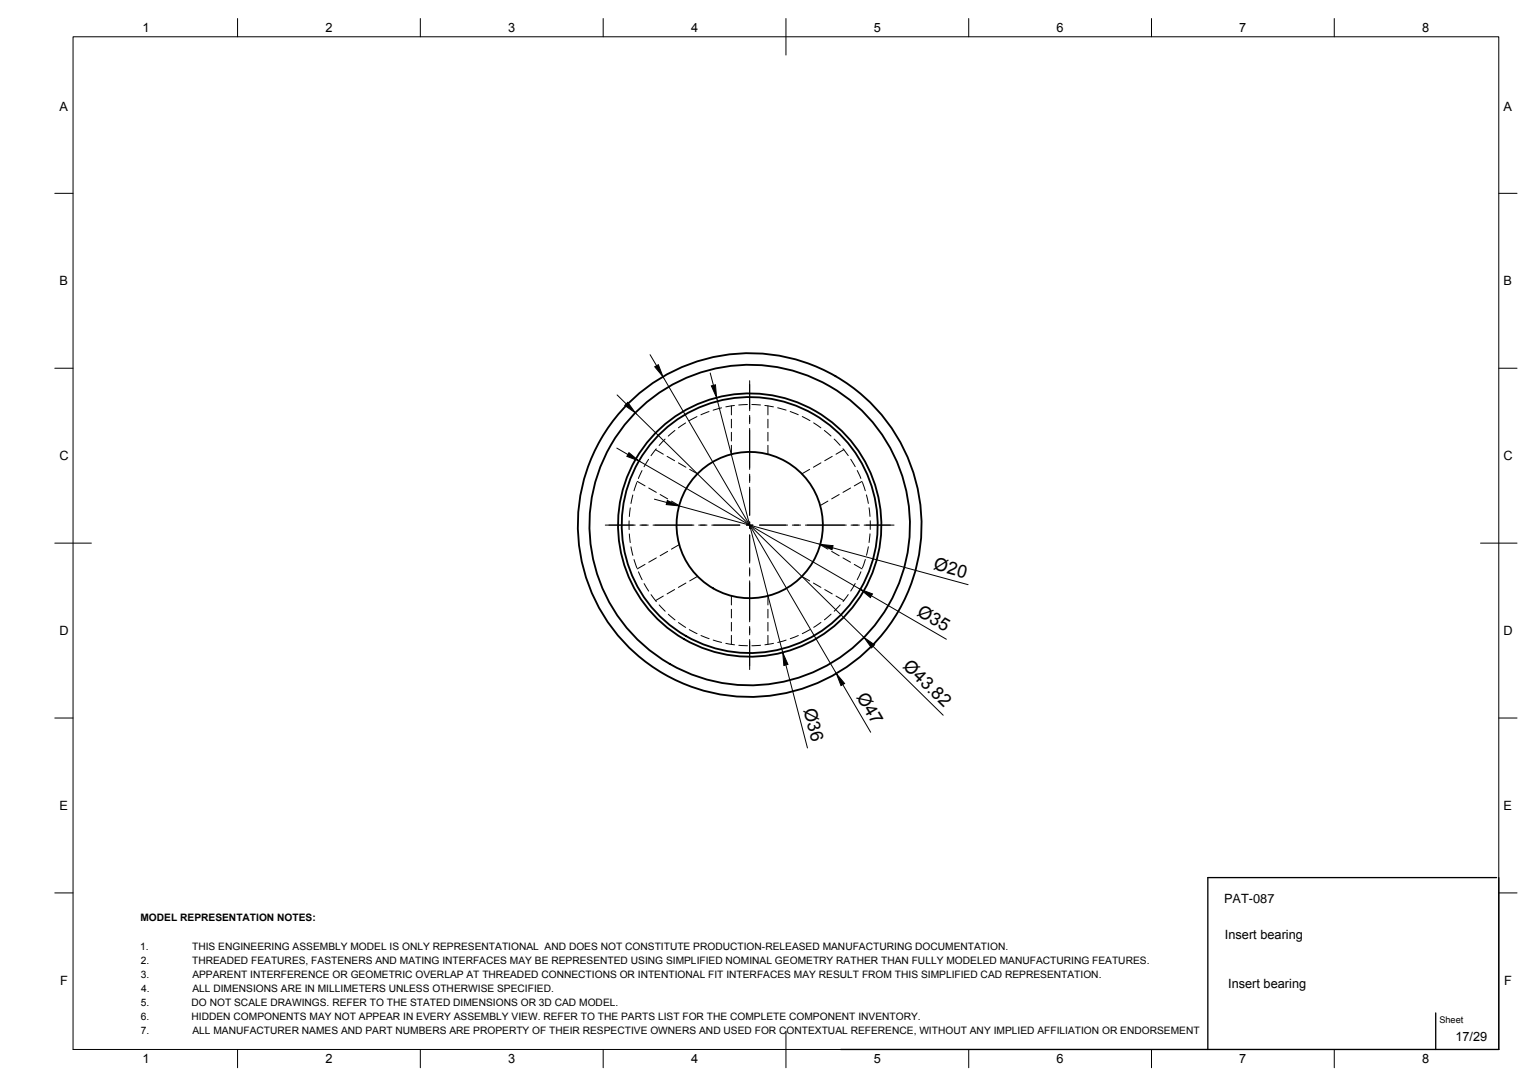
ISO-10303-21;
HEADER;
/* Generated by software containing ST-Developer
 * from STEP Tools, Inc. (www.steptools.com) 
 */

FILE_DESCRIPTION(
/* description */ ('Rigid flange shaft coupling assembly'),
/* implementation_level */ '2;1');

FILE_NAME(
/* name */ 'Insert bearing.step',
/* time_stamp */ '2026-10-27T10:47:16-07:00',
/* author */ (''),
/* organization */ (''),
/* preprocessor_version */ 'ST-DEVELOPER v20.2',
/* originating_system */ 'Autodesk Translation Framework v15.17.0.0',
/* authorisation */ '');

FILE_SCHEMA (('AUTOMOTIVE_DESIGN { 1 0 10303 214 3 1 1 }'));
ENDSEC;

DATA;
#10=MECHANICAL_DESIGN_GEOMETRIC_PRESENTATION_REPRESENTATION('',(#408,#409),#9141);
#300=B_SPLINE_CURVE_WITH_KNOTS('',3,(#7504,#7505,#7506,#7507,#7508,#7509,
#7510,#7511,#7512,#7513),.UNSPECIFIED.,.F.,.F.,(4,2,2,2,4),(1.13193471301885,
1.22626174930539,1.32058878559194,1.41491753480854,1.50924628402513),
 .UNSPECIFIED.);
#301=B_SPLINE_CURVE_WITH_KNOTS('',3,(#7515,#7516,#7517,#7518,#7519,#7520,
#7521,#7522,#7523,#7524,#7525,#7526,#7527,#7528,#7529,#7530,#7531,#7532),
 .UNSPECIFIED.,.F.,.F.,(4,2,2,2,2,2,2,2,4),(0.377311571006283,0.471638607292829,
0.565965643579376,0.66029439279597,0.754623142012565,0.84895189122916,0.943280640445754,
1.0376076767323,1.13193471301885),.UNSPECIFIED.);
#302=B_SPLINE_CURVE_WITH_KNOTS('',3,(#7533,#7534,#7535,#7536,#7537,#7538,
#7539,#7540,#7541,#7542),.UNSPECIFIED.,.F.,.F.,(4,2,2,2,4),(1.50924628402513,
1.60357503324173,1.69790378245832,1.79223081874487,1.88655785503141),
 .UNSPECIFIED.);
#303=B_SPLINE_CURVE_WITH_KNOTS('',3,(#7545,#7546,#7547,#7548,#7549,#7550,
#7551,#7552,#7553,#7554,#7555,#7556,#7557,#7558,#7559,#7560,#7561,#7562,
#7563,#7564,#7565,#7566,#7567,#7568,#7569,#7570,#7571,#7572,#7573,#7574,
#7575,#7576,#7577,#7578),.UNSPECIFIED.,.T.,.F.,(4,2,2,2,2,2,2,2,2,2,2,2,
2,2,2,2,4),(0.,0.0946120580087934,0.189224116017587,0.283822945575014,0.378421775132442,
0.47302060468987,0.567619434247297,0.662231492256091,0.756843550264884,
0.851455608273677,0.94606766628247,1.0406664958399,1.13526532539733,1.22986415495475,
1.32446298451218,1.41907504252097,1.51368710052977),.UNSPECIFIED.);
#304=B_SPLINE_CURVE_WITH_KNOTS('',3,(#7581,#7582,#7583,#7584,#7585,#7586,
#7587,#7588,#7589,#7590,#7591,#7592,#7593,#7594,#7595,#7596,#7597,#7598,
#7599,#7600,#7601,#7602,#7603,#7604,#7605,#7606,#7607,#7608,#7609,#7610,
#7611,#7612,#7613,#7614),.UNSPECIFIED.,.T.,.F.,(4,2,2,2,2,2,2,2,2,2,2,2,
2,2,2,2,4),(0.,0.0946120580087934,0.189224116017587,0.283822945575014,0.378421775132442,
0.47302060468987,0.567619434247297,0.66223149225609,0.756843550264884,0.851455608273677,
0.94606766628247,1.0406664958399,1.13526532539733,1.22986415495475,1.32446298451218,
1.41907504252097,1.51368710052977),.UNSPECIFIED.);
#305=B_SPLINE_CURVE_WITH_KNOTS('',3,(#7618,#7619,#7620,#7621,#7622,#7623,
#7624,#7625,#7626,#7627),.UNSPECIFIED.,.F.,.F.,(4,2,2,2,4),(1.13193471301885,
1.22626174930539,1.32058878559194,1.41491753480854,1.50924628402513),
 .UNSPECIFIED.);
#306=B_SPLINE_CURVE_WITH_KNOTS('',3,(#7629,#7630,#7631,#7632,#7633,#7634,
#7635,#7636,#7637,#7638,#7639,#7640,#7641,#7642,#7643,#7644,#7645,#7646),
 .UNSPECIFIED.,.F.,.F.,(4,2,2,2,2,2,2,2,4),(0.377311571006283,0.47163860729283,
0.565965643579376,0.660294392795971,0.754623142012565,0.84895189122916,
0.943280640445755,1.0376076767323,1.13193471301885),.UNSPECIFIED.);
#307=B_SPLINE_CURVE_WITH_KNOTS('',3,(#7647,#7648,#7649,#7650,#7651,#7652,
#7653,#7654,#7655,#7656),.UNSPECIFIED.,.F.,.F.,(4,2,2,2,4),(1.50924628402513,
1.60357503324173,1.69790378245832,1.79223081874487,1.88655785503141),
 .UNSPECIFIED.);
#308=B_SPLINE_CURVE_WITH_KNOTS('',3,(#7665,#7666,#7667,#7668,#7669,#7670,
#7671,#7672,#7673,#7674,#7675,#7676,#7677,#7678,#7679,#7680,#7681,#7682),
 .UNSPECIFIED.,.F.,.F.,(4,2,2,2,2,2,2,2,4),(0.377311571006282,0.471638607292829,
0.565965643579376,0.660294392795971,0.754623142012565,0.84895189122916,
0.943280640445754,1.0376076767323,1.13193471301885),.UNSPECIFIED.);
#309=B_SPLINE_CURVE_WITH_KNOTS('',3,(#7684,#7685,#7686,#7687,#7688,#7689,
#7690,#7691,#7692,#7693),.UNSPECIFIED.,.F.,.F.,(4,2,2,2,4),(1.13193471301885,
1.22626174930539,1.32058878559194,1.41491753480854,1.50924628402513),
 .UNSPECIFIED.);
#310=B_SPLINE_CURVE_WITH_KNOTS('',3,(#7694,#7695,#7696,#7697,#7698,#7699,
#7700,#7701,#7702,#7703),.UNSPECIFIED.,.F.,.F.,(4,2,2,2,4),(1.50924628402513,
1.60357503324172,1.69790378245832,1.79223081874487,1.88655785503141),
 .UNSPECIFIED.);
#311=B_SPLINE_CURVE_WITH_KNOTS('',3,(#7706,#7707,#7708,#7709,#7710,#7711,
#7712,#7713,#7714,#7715,#7716,#7717,#7718,#7719,#7720,#7721,#7722,#7723),
 .UNSPECIFIED.,.F.,.F.,(4,2,2,2,2,2,2,2,4),(0.377311571006283,0.47163860729283,
0.565965643579376,0.660294392795971,0.754623142012565,0.84895189122916,
0.943280640445754,1.0376076767323,1.13193471301885),.UNSPECIFIED.);
#312=B_SPLINE_CURVE_WITH_KNOTS('',3,(#7725,#7726,#7727,#7728,#7729,#7730,
#7731,#7732,#7733,#7734),.UNSPECIFIED.,.F.,.F.,(4,2,2,2,4),(1.13193471301885,
1.22626174930539,1.32058878559194,1.41491753480854,1.50924628402513),
 .UNSPECIFIED.);
#313=B_SPLINE_CURVE_WITH_KNOTS('',3,(#7735,#7736,#7737,#7738,#7739,#7740,
#7741,#7742,#7743,#7744),.UNSPECIFIED.,.F.,.F.,(4,2,2,2,4),(1.50924628402513,
1.60357503324173,1.69790378245832,1.79223081874487,1.88655785503141),
 .UNSPECIFIED.);
#314=B_SPLINE_CURVE_WITH_KNOTS('',3,(#7747,#7748,#7749,#7750,#7751,#7752,
#7753,#7754,#7755,#7756,#7757,#7758,#7759,#7760,#7761,#7762,#7763,#7764),
 .UNSPECIFIED.,.F.,.F.,(4,2,2,2,2,2,2,2,4),(0.377311571006282,0.471638607292829,
0.565965643579376,0.66029439279597,0.754623142012565,0.84895189122916,0.943280640445754,
1.0376076767323,1.13193471301885),.UNSPECIFIED.);
#315=B_SPLINE_CURVE_WITH_KNOTS('',3,(#7766,#7767,#7768,#7769,#7770,#7771,
#7772,#7773,#7774,#7775),.UNSPECIFIED.,.F.,.F.,(4,2,2,2,4),(1.13193471301885,
1.22626174930539,1.32058878559194,1.41491753480854,1.50924628402513),
 .UNSPECIFIED.);
#316=B_SPLINE_CURVE_WITH_KNOTS('',3,(#7776,#7777,#7778,#7779,#7780,#7781,
#7782,#7783,#7784,#7785),.UNSPECIFIED.,.F.,.F.,(4,2,2,2,4),(1.50924628402513,
1.60357503324172,1.69790378245832,1.79223081874487,1.88655785503141),
 .UNSPECIFIED.);
#317=B_SPLINE_CURVE_WITH_KNOTS('',3,(#7788,#7789,#7790,#7791,#7792,#7793,
#7794,#7795,#7796,#7797,#7798,#7799,#7800,#7801,#7802,#7803,#7804,#7805),
 .UNSPECIFIED.,.F.,.F.,(4,2,2,2,2,2,2,2,4),(0.377311571006283,0.471638607292829,
0.565965643579376,0.660294392795971,0.754623142012565,0.84895189122916,
0.943280640445755,1.0376076767323,1.13193471301885),.UNSPECIFIED.);
#318=B_SPLINE_CURVE_WITH_KNOTS('',3,(#7807,#7808,#7809,#7810,#7811,#7812,
#7813,#7814,#7815,#7816),.UNSPECIFIED.,.F.,.F.,(4,2,2,2,4),(1.13193471301885,
1.22626174930539,1.32058878559194,1.41491753480854,1.50924628402513),
 .UNSPECIFIED.);
#319=B_SPLINE_CURVE_WITH_KNOTS('',3,(#7817,#7818,#7819,#7820,#7821,#7822,
#7823,#7824,#7825,#7826),.UNSPECIFIED.,.F.,.F.,(4,2,2,2,4),(1.50924628402513,
1.60357503324172,1.69790378245832,1.79223081874487,1.88655785503141),
 .UNSPECIFIED.);
#320=B_SPLINE_CURVE_WITH_KNOTS('',3,(#7830,#7831,#7832,#7833,#7834,#7835,
#7836,#7837,#7838,#7839,#7840,#7841,#7842,#7843,#7844,#7845,#7846,#7847,
#7848,#7849,#7850,#7851,#7852,#7853,#7854,#7855,#7856,#7857,#7858,#7859,
#7860,#7861,#7862,#7863),.UNSPECIFIED.,.T.,.F.,(4,2,2,2,2,2,2,2,2,2,2,2,
2,2,2,2,4),(0.,0.0946120580087934,0.189224116017587,0.283822945575014,0.378421775132442,
0.47302060468987,0.567619434247297,0.66223149225609,0.756843550264884,0.851455608273677,
0.94606766628247,1.0406664958399,1.13526532539733,1.22986415495475,1.32446298451218,
1.41907504252097,1.51368710052977),.UNSPECIFIED.);
#321=B_SPLINE_CURVE_WITH_KNOTS('',3,(#7866,#7867,#7868,#7869,#7870,#7871,
#7872,#7873,#7874,#7875,#7876,#7877,#7878,#7879,#7880,#7881,#7882,#7883,
#7884,#7885,#7886,#7887,#7888,#7889,#7890,#7891,#7892,#7893,#7894,#7895,
#7896,#7897,#7898,#7899),.UNSPECIFIED.,.T.,.F.,(4,2,2,2,2,2,2,2,2,2,2,2,
2,2,2,2,4),(0.,0.0946120580087934,0.189224116017587,0.283822945575014,0.378421775132442,
0.47302060468987,0.567619434247297,0.66223149225609,0.756843550264884,0.851455608273677,
0.94606766628247,1.0406664958399,1.13526532539733,1.22986415495475,1.32446298451218,
1.41907504252097,1.51368710052977),.UNSPECIFIED.);
#322=B_SPLINE_CURVE_WITH_KNOTS('',3,(#7904,#7905,#7906,#7907,#7908,#7909,
#7910,#7911,#7912,#7913,#7914,#7915,#7916,#7917,#7918,#7919,#7920,#7921,
#7922,#7923,#7924,#7925,#7926,#7927,#7928,#7929,#7930,#7931,#7932,#7933,
#7934,#7935,#7936,#7937),.UNSPECIFIED.,.T.,.F.,(4,2,2,2,2,2,2,2,2,2,2,2,
2,2,2,2,4),(0.,0.0946120580087934,0.189224116017587,0.283822945575014,0.378421775132442,
0.47302060468987,0.567619434247297,0.66223149225609,0.756843550264884,0.851455608273677,
0.94606766628247,1.0406664958399,1.13526532539733,1.22986415495475,1.32446298451218,
1.41907504252097,1.51368710052977),.UNSPECIFIED.);
#323=B_SPLINE_CURVE_WITH_KNOTS('',3,(#7940,#7941,#7942,#7943,#7944,#7945,
#7946,#7947,#7948,#7949,#7950,#7951,#7952,#7953,#7954,#7955,#7956,#7957,
#7958,#7959,#7960,#7961,#7962,#7963,#7964,#7965,#7966,#7967,#7968,#7969,
#7970,#7971,#7972,#7973),.UNSPECIFIED.,.T.,.F.,(4,2,2,2,2,2,2,2,2,2,2,2,
2,2,2,2,4),(0.,0.0946120580087934,0.189224116017587,0.283822945575014,0.378421775132442,
0.47302060468987,0.567619434247297,0.66223149225609,0.756843550264884,0.851455608273677,
0.94606766628247,1.0406664958399,1.13526532539733,1.22986415495475,1.32446298451218,
1.41907504252097,1.51368710052977),.UNSPECIFIED.);
#341=SPHERICAL_SURFACE('',#5250,2.35);
#352=SHAPE_REPRESENTATION_RELATIONSHIP('SRR','None',#9287,#380);
#380=ADVANCED_BREP_SHAPE_REPRESENTATION('',(#437,#438),#9122);
#408=STYLED_ITEM('',(#9500),#437);
#409=STYLED_ITEM('',(#9500),#438);
#437=MANIFOLD_SOLID_BREP('Body1',#4762);
#438=MANIFOLD_SOLID_BREP('Body2',#4763);
#495=FACE_BOUND('',#1143,.T.);
#496=FACE_BOUND('',#1145,.T.);
#497=FACE_BOUND('',#1146,.T.);
#498=FACE_BOUND('',#1148,.T.);
#499=FACE_BOUND('',#1152,.T.);
#500=FACE_BOUND('',#1153,.T.);
#501=FACE_BOUND('',#1154,.T.);
#502=FACE_BOUND('',#1155,.T.);
#503=FACE_BOUND('',#1156,.T.);
#504=FACE_BOUND('',#1157,.T.);
#505=FACE_BOUND('',#1163,.T.);
#506=FACE_BOUND('',#1165,.T.);
#507=FACE_BOUND('',#1168,.T.);
#508=FACE_BOUND('',#1170,.T.);
#509=FACE_BOUND('',#1171,.T.);
#510=FACE_BOUND('',#1172,.T.);
#511=FACE_BOUND('',#1173,.T.);
#512=FACE_BOUND('',#1174,.T.);
#513=FACE_BOUND('',#1175,.T.);
#627=PLANE('',#5248);
#628=PLANE('',#5253);
#629=PLANE('',#5263);
#630=PLANE('',#5265);
#631=PLANE('',#5269);
#827=FACE_OUTER_BOUND('',#1141,.T.);
#828=FACE_OUTER_BOUND('',#1142,.T.);
#829=FACE_OUTER_BOUND('',#1144,.T.);
#830=FACE_OUTER_BOUND('',#1147,.T.);
#831=FACE_OUTER_BOUND('',#1149,.T.);
#832=FACE_OUTER_BOUND('',#1150,.T.);
#833=FACE_OUTER_BOUND('',#1151,.T.);
#834=FACE_OUTER_BOUND('',#1158,.T.);
#835=FACE_OUTER_BOUND('',#1159,.T.);
#836=FACE_OUTER_BOUND('',#1160,.T.);
#837=FACE_OUTER_BOUND('',#1161,.T.);
#838=FACE_OUTER_BOUND('',#1162,.T.);
#839=FACE_OUTER_BOUND('',#1164,.T.);
#840=FACE_OUTER_BOUND('',#1166,.T.);
#841=FACE_OUTER_BOUND('',#1167,.T.);
#842=FACE_OUTER_BOUND('',#1169,.T.);
#1141=EDGE_LOOP('',(#3605,#3606,#3607,#3608));
#1142=EDGE_LOOP('',(#3609));
#1143=EDGE_LOOP('',(#3610));
#1144=EDGE_LOOP('',(#3611,#3612));
#1145=EDGE_LOOP('',(#3613));
#1146=EDGE_LOOP('',(#3614));
#1147=EDGE_LOOP('',(#3615));
#1148=EDGE_LOOP('',(#3616));
#1149=EDGE_LOOP('',(#3617,#3618,#3619,#3620,#3621,#3622));
#1150=EDGE_LOOP('',(#3623,#3624,#3625,#3626,#3627,#3628));
#1151=EDGE_LOOP('',(#3629,#3630,#3631,#3632));
#1152=EDGE_LOOP('',(#3633,#3634,#3635));
#1153=EDGE_LOOP('',(#3636,#3637,#3638));
#1154=EDGE_LOOP('',(#3639,#3640,#3641));
#1155=EDGE_LOOP('',(#3642,#3643,#3644));
#1156=EDGE_LOOP('',(#3645,#3646,#3647));
#1157=EDGE_LOOP('',(#3648,#3649,#3650));
#1158=EDGE_LOOP('',(#3651,#3652,#3653,#3654,#3655,#3656));
#1159=EDGE_LOOP('',(#3657,#3658,#3659,#3660,#3661,#3662));
#1160=EDGE_LOOP('',(#3663,#3664,#3665,#3666,#3667,#3668));
#1161=EDGE_LOOP('',(#3669,#3670,#3671,#3672,#3673,#3674));
#1162=EDGE_LOOP('',(#3675));
#1163=EDGE_LOOP('',(#3676));
#1164=EDGE_LOOP('',(#3677));
#1165=EDGE_LOOP('',(#3678));
#1166=EDGE_LOOP('',(#3679,#3680,#3681,#3682));
#1167=EDGE_LOOP('',(#3683));
#1168=EDGE_LOOP('',(#3684));
#1169=EDGE_LOOP('',(#3685,#3686,#3687,#3688));
#1170=EDGE_LOOP('',(#3689));
#1171=EDGE_LOOP('',(#3690));
#1172=EDGE_LOOP('',(#3691));
#1173=EDGE_LOOP('',(#3692));
#1174=EDGE_LOOP('',(#3693));
#1175=EDGE_LOOP('',(#3694));
#1531=LINE('',#7489,#1876);
#1532=LINE('',#7544,#1877);
#1533=LINE('',#7616,#1878);
#1534=LINE('',#7661,#1879);
#1535=LINE('',#7829,#1880);
#1536=LINE('',#7900,#1881);
#1537=LINE('',#7903,#1882);
#1538=LINE('',#7974,#1883);
#1539=LINE('',#7984,#1884);
#1540=LINE('',#7989,#1885);
#1876=VECTOR('',#6076,1.8);
#1877=VECTOR('',#6093,0.25);
#1878=VECTOR('',#6096,0.25);
#1879=VECTOR('',#6101,1.65);
#1880=VECTOR('',#6106,0.25);
#1881=VECTOR('',#6109,0.25);
#1882=VECTOR('',#6112,0.25);
#1883=VECTOR('',#6115,0.25);
#1884=VECTOR('',#6128,1.75);
#1885=VECTOR('',#6135,1.);
#2150=CIRCLE('',#5246,1.8);
#2151=CIRCLE('',#5247,1.8);
#2152=CIRCLE('',#5249,2.19089023002066);
#2153=CIRCLE('',#5251,2.35);
#2154=CIRCLE('',#5252,2.19089023002066);
#2155=CIRCLE('',#5257,1.65);
#2156=CIRCLE('',#5258,1.65);
#2157=CIRCLE('',#5264,1.);
#2158=CIRCLE('',#5266,1.75);
#2159=CIRCLE('',#5268,1.75);
#2160=CIRCLE('',#5270,1.);
#2398=VERTEX_POINT('',#7486);
#2399=VERTEX_POINT('',#7488);
#2400=VERTEX_POINT('',#7492);
#2401=VERTEX_POINT('',#7495);
#2402=VERTEX_POINT('',#7496);
#2403=VERTEX_POINT('',#7498);
#2404=VERTEX_POINT('',#7502);
#2405=VERTEX_POINT('',#7503);
#2406=VERTEX_POINT('',#7514);
#2407=VERTEX_POINT('',#7543);
#2408=VERTEX_POINT('',#7580);
#2409=VERTEX_POINT('',#7615);
#2410=VERTEX_POINT('',#7617);
#2411=VERTEX_POINT('',#7628);
#2412=VERTEX_POINT('',#7658);
#2413=VERTEX_POINT('',#7660);
#2414=VERTEX_POINT('',#7663);
#2415=VERTEX_POINT('',#7664);
#2416=VERTEX_POINT('',#7683);
#2417=VERTEX_POINT('',#7704);
#2418=VERTEX_POINT('',#7705);
#2419=VERTEX_POINT('',#7724);
#2420=VERTEX_POINT('',#7745);
#2421=VERTEX_POINT('',#7746);
#2422=VERTEX_POINT('',#7765);
#2423=VERTEX_POINT('',#7786);
#2424=VERTEX_POINT('',#7787);
#2425=VERTEX_POINT('',#7806);
#2426=VERTEX_POINT('',#7828);
#2427=VERTEX_POINT('',#7865);
#2428=VERTEX_POINT('',#7902);
#2429=VERTEX_POINT('',#7939);
#2430=VERTEX_POINT('',#7976);
#2431=VERTEX_POINT('',#7979);
#2432=VERTEX_POINT('',#7982);
#2433=VERTEX_POINT('',#7986);
#2846=EDGE_CURVE('',#2398,#2398,#2150,.T.);
#2847=EDGE_CURVE('',#2398,#2399,#1531,.T.);
#2848=EDGE_CURVE('',#2399,#2399,#2151,.T.);
#2849=EDGE_CURVE('',#2400,#2400,#2152,.T.);
#2850=EDGE_CURVE('',#2401,#2402,#2153,.T.);
#2851=EDGE_CURVE('',#2403,#2403,#2154,.T.);
#2852=EDGE_CURVE('',#2404,#2405,#300,.T.);
#2853=EDGE_CURVE('',#2406,#2404,#301,.T.);
#2854=EDGE_CURVE('',#2405,#2406,#302,.T.);
#2855=EDGE_CURVE('',#2405,#2407,#1532,.T.);
#2856=EDGE_CURVE('',#2407,#2407,#303,.T.);
#2857=EDGE_CURVE('',#2408,#2408,#304,.T.);
#2858=EDGE_CURVE('',#2408,#2409,#1533,.T.);
#2859=EDGE_CURVE('',#2410,#2409,#305,.T.);
#2860=EDGE_CURVE('',#2411,#2410,#306,.T.);
#2861=EDGE_CURVE('',#2409,#2411,#307,.T.);
#2862=EDGE_CURVE('',#2412,#2412,#2155,.T.);
#2863=EDGE_CURVE('',#2412,#2413,#1534,.T.);
#2864=EDGE_CURVE('',#2413,#2413,#2156,.T.);
#2865=EDGE_CURVE('',#2414,#2415,#308,.T.);
#2866=EDGE_CURVE('',#2415,#2416,#309,.T.);
#2867=EDGE_CURVE('',#2416,#2414,#310,.T.);
#2868=EDGE_CURVE('',#2417,#2418,#311,.T.);
#2869=EDGE_CURVE('',#2418,#2419,#312,.T.);
#2870=EDGE_CURVE('',#2419,#2417,#313,.T.);
#2871=EDGE_CURVE('',#2420,#2421,#314,.T.);
#2872=EDGE_CURVE('',#2421,#2422,#315,.T.);
#2873=EDGE_CURVE('',#2422,#2420,#316,.T.);
#2874=EDGE_CURVE('',#2423,#2424,#317,.T.);
#2875=EDGE_CURVE('',#2424,#2425,#318,.T.);
#2876=EDGE_CURVE('',#2425,#2423,#319,.T.);
#2877=EDGE_CURVE('',#2416,#2426,#1535,.T.);
#2878=EDGE_CURVE('',#2426,#2426,#320,.T.);
#2879=EDGE_CURVE('',#2427,#2427,#321,.T.);
#2880=EDGE_CURVE('',#2427,#2419,#1536,.T.);
#2881=EDGE_CURVE('',#2422,#2428,#1537,.T.);
#2882=EDGE_CURVE('',#2428,#2428,#322,.T.);
#2883=EDGE_CURVE('',#2429,#2429,#323,.T.);
#2884=EDGE_CURVE('',#2429,#2425,#1538,.T.);
#2885=EDGE_CURVE('',#2430,#2430,#2157,.T.);
#2886=EDGE_CURVE('',#2431,#2431,#2158,.T.);
#2887=EDGE_CURVE('',#2432,#2432,#2159,.T.);
#2888=EDGE_CURVE('',#2432,#2431,#1539,.T.);
#2889=EDGE_CURVE('',#2433,#2433,#2160,.T.);
#2890=EDGE_CURVE('',#2433,#2430,#1540,.T.);
#3605=ORIENTED_EDGE('',*,*,#2846,.T.);
#3606=ORIENTED_EDGE('',*,*,#2847,.T.);
#3607=ORIENTED_EDGE('',*,*,#2848,.F.);
#3608=ORIENTED_EDGE('',*,*,#2847,.F.);
#3609=ORIENTED_EDGE('',*,*,#2849,.F.);
#3610=ORIENTED_EDGE('',*,*,#2848,.T.);
#3611=ORIENTED_EDGE('',*,*,#2850,.T.);
#3612=ORIENTED_EDGE('',*,*,#2850,.F.);
#3613=ORIENTED_EDGE('',*,*,#2849,.T.);
#3614=ORIENTED_EDGE('',*,*,#2851,.F.);
#3615=ORIENTED_EDGE('',*,*,#2851,.T.);
#3616=ORIENTED_EDGE('',*,*,#2846,.F.);
#3617=ORIENTED_EDGE('',*,*,#2852,.F.);
#3618=ORIENTED_EDGE('',*,*,#2853,.F.);
#3619=ORIENTED_EDGE('',*,*,#2854,.F.);
#3620=ORIENTED_EDGE('',*,*,#2855,.T.);
#3621=ORIENTED_EDGE('',*,*,#2856,.F.);
#3622=ORIENTED_EDGE('',*,*,#2855,.F.);
#3623=ORIENTED_EDGE('',*,*,#2857,.F.);
#3624=ORIENTED_EDGE('',*,*,#2858,.T.);
#3625=ORIENTED_EDGE('',*,*,#2859,.F.);
#3626=ORIENTED_EDGE('',*,*,#2860,.F.);
#3627=ORIENTED_EDGE('',*,*,#2861,.F.);
#3628=ORIENTED_EDGE('',*,*,#2858,.F.);
#3629=ORIENTED_EDGE('',*,*,#2862,.F.);
#3630=ORIENTED_EDGE('',*,*,#2863,.T.);
#3631=ORIENTED_EDGE('',*,*,#2864,.T.);
#3632=ORIENTED_EDGE('',*,*,#2863,.F.);
#3633=ORIENTED_EDGE('',*,*,#2853,.T.);
#3634=ORIENTED_EDGE('',*,*,#2852,.T.);
#3635=ORIENTED_EDGE('',*,*,#2854,.T.);
#3636=ORIENTED_EDGE('',*,*,#2860,.T.);
#3637=ORIENTED_EDGE('',*,*,#2859,.T.);
#3638=ORIENTED_EDGE('',*,*,#2861,.T.);
#3639=ORIENTED_EDGE('',*,*,#2865,.T.);
#3640=ORIENTED_EDGE('',*,*,#2866,.T.);
#3641=ORIENTED_EDGE('',*,*,#2867,.T.);
#3642=ORIENTED_EDGE('',*,*,#2868,.T.);
#3643=ORIENTED_EDGE('',*,*,#2869,.T.);
#3644=ORIENTED_EDGE('',*,*,#2870,.T.);
#3645=ORIENTED_EDGE('',*,*,#2871,.T.);
#3646=ORIENTED_EDGE('',*,*,#2872,.T.);
#3647=ORIENTED_EDGE('',*,*,#2873,.T.);
#3648=ORIENTED_EDGE('',*,*,#2874,.T.);
#3649=ORIENTED_EDGE('',*,*,#2875,.T.);
#3650=ORIENTED_EDGE('',*,*,#2876,.T.);
#3651=ORIENTED_EDGE('',*,*,#2866,.F.);
#3652=ORIENTED_EDGE('',*,*,#2865,.F.);
#3653=ORIENTED_EDGE('',*,*,#2867,.F.);
#3654=ORIENTED_EDGE('',*,*,#2877,.T.);
#3655=ORIENTED_EDGE('',*,*,#2878,.F.);
#3656=ORIENTED_EDGE('',*,*,#2877,.F.);
#3657=ORIENTED_EDGE('',*,*,#2879,.F.);
#3658=ORIENTED_EDGE('',*,*,#2880,.T.);
#3659=ORIENTED_EDGE('',*,*,#2869,.F.);
#3660=ORIENTED_EDGE('',*,*,#2868,.F.);
#3661=ORIENTED_EDGE('',*,*,#2870,.F.);
#3662=ORIENTED_EDGE('',*,*,#2880,.F.);
#3663=ORIENTED_EDGE('',*,*,#2872,.F.);
#3664=ORIENTED_EDGE('',*,*,#2871,.F.);
#3665=ORIENTED_EDGE('',*,*,#2873,.F.);
#3666=ORIENTED_EDGE('',*,*,#2881,.T.);
#3667=ORIENTED_EDGE('',*,*,#2882,.F.);
#3668=ORIENTED_EDGE('',*,*,#2881,.F.);
#3669=ORIENTED_EDGE('',*,*,#2883,.F.);
#3670=ORIENTED_EDGE('',*,*,#2884,.T.);
#3671=ORIENTED_EDGE('',*,*,#2875,.F.);
#3672=ORIENTED_EDGE('',*,*,#2874,.F.);
#3673=ORIENTED_EDGE('',*,*,#2876,.F.);
#3674=ORIENTED_EDGE('',*,*,#2884,.F.);
#3675=ORIENTED_EDGE('',*,*,#2864,.F.);
#3676=ORIENTED_EDGE('',*,*,#2885,.T.);
#3677=ORIENTED_EDGE('',*,*,#2886,.F.);
#3678=ORIENTED_EDGE('',*,*,#2862,.T.);
#3679=ORIENTED_EDGE('',*,*,#2887,.F.);
#3680=ORIENTED_EDGE('',*,*,#2888,.T.);
#3681=ORIENTED_EDGE('',*,*,#2886,.T.);
#3682=ORIENTED_EDGE('',*,*,#2888,.F.);
#3683=ORIENTED_EDGE('',*,*,#2887,.T.);
#3684=ORIENTED_EDGE('',*,*,#2889,.F.);
#3685=ORIENTED_EDGE('',*,*,#2889,.T.);
#3686=ORIENTED_EDGE('',*,*,#2890,.T.);
#3687=ORIENTED_EDGE('',*,*,#2885,.F.);
#3688=ORIENTED_EDGE('',*,*,#2890,.F.);
#3689=ORIENTED_EDGE('',*,*,#2857,.T.);
#3690=ORIENTED_EDGE('',*,*,#2856,.T.);
#3691=ORIENTED_EDGE('',*,*,#2879,.T.);
#3692=ORIENTED_EDGE('',*,*,#2878,.T.);
#3693=ORIENTED_EDGE('',*,*,#2883,.T.);
#3694=ORIENTED_EDGE('',*,*,#2882,.T.);
#4424=CYLINDRICAL_SURFACE('',#5245,1.8);
#4425=CYLINDRICAL_SURFACE('',#5254,0.25);
#4426=CYLINDRICAL_SURFACE('',#5255,0.25);
#4427=CYLINDRICAL_SURFACE('',#5256,1.65);
#4428=CYLINDRICAL_SURFACE('',#5259,0.25);
#4429=CYLINDRICAL_SURFACE('',#5260,0.25);
#4430=CYLINDRICAL_SURFACE('',#5261,0.25);
#4431=CYLINDRICAL_SURFACE('',#5262,0.25);
#4432=CYLINDRICAL_SURFACE('',#5267,1.75);
#4433=CYLINDRICAL_SURFACE('',#5271,1.);
#4563=ADVANCED_FACE('',(#827),#4424,.F.);
#4564=ADVANCED_FACE('',(#828,#495),#627,.T.);
#4565=ADVANCED_FACE('',(#829,#496,#497),#341,.T.);
#4566=ADVANCED_FACE('',(#830,#498),#628,.T.);
#4567=ADVANCED_FACE('',(#831),#4425,.F.);
#4568=ADVANCED_FACE('',(#832),#4426,.F.);
#4569=ADVANCED_FACE('',(#833,#499,#500,#501,#502,#503,#504),#4427,.T.);
#4570=ADVANCED_FACE('',(#834),#4428,.F.);
#4571=ADVANCED_FACE('',(#835),#4429,.F.);
#4572=ADVANCED_FACE('',(#836),#4430,.F.);
#4573=ADVANCED_FACE('',(#837),#4431,.F.);
#4574=ADVANCED_FACE('',(#838,#505),#629,.T.);
#4575=ADVANCED_FACE('',(#839,#506),#630,.T.);
#4576=ADVANCED_FACE('',(#840),#4432,.T.);
#4577=ADVANCED_FACE('',(#841,#507),#631,.T.);
#4578=ADVANCED_FACE('',(#842,#508,#509,#510,#511,#512,#513),#4433,.F.);
#4762=CLOSED_SHELL('',(#4563,#4564,#4565,#4566));
#4763=CLOSED_SHELL('',(#4567,#4568,#4569,#4570,#4571,#4572,#4573,#4574,
#4575,#4576,#4577,#4578));
#5244=AXIS2_PLACEMENT_3D('',#7484,#6070,#6071);
#5245=AXIS2_PLACEMENT_3D('',#7485,#6072,#6073);
#5246=AXIS2_PLACEMENT_3D('',#7487,#6074,#6075);
#5247=AXIS2_PLACEMENT_3D('',#7490,#6077,#6078);
#5248=AXIS2_PLACEMENT_3D('',#7491,#6079,#6080);
#5249=AXIS2_PLACEMENT_3D('',#7493,#6081,#6082);
#5250=AXIS2_PLACEMENT_3D('',#7494,#6083,#6084);
#5251=AXIS2_PLACEMENT_3D('',#7497,#6085,#6086);
#5252=AXIS2_PLACEMENT_3D('',#7499,#6087,#6088);
#5253=AXIS2_PLACEMENT_3D('',#7500,#6089,#6090);
#5254=AXIS2_PLACEMENT_3D('',#7501,#6091,#6092);
#5255=AXIS2_PLACEMENT_3D('',#7579,#6094,#6095);
#5256=AXIS2_PLACEMENT_3D('',#7657,#6097,#6098);
#5257=AXIS2_PLACEMENT_3D('',#7659,#6099,#6100);
#5258=AXIS2_PLACEMENT_3D('',#7662,#6102,#6103);
#5259=AXIS2_PLACEMENT_3D('',#7827,#6104,#6105);
#5260=AXIS2_PLACEMENT_3D('',#7864,#6107,#6108);
#5261=AXIS2_PLACEMENT_3D('',#7901,#6110,#6111);
#5262=AXIS2_PLACEMENT_3D('',#7938,#6113,#6114);
#5263=AXIS2_PLACEMENT_3D('',#7975,#6116,#6117);
#5264=AXIS2_PLACEMENT_3D('',#7977,#6118,#6119);
#5265=AXIS2_PLACEMENT_3D('',#7978,#6120,#6121);
#5266=AXIS2_PLACEMENT_3D('',#7980,#6122,#6123);
#5267=AXIS2_PLACEMENT_3D('',#7981,#6124,#6125);
#5268=AXIS2_PLACEMENT_3D('',#7983,#6126,#6127);
#5269=AXIS2_PLACEMENT_3D('',#7985,#6129,#6130);
#5270=AXIS2_PLACEMENT_3D('',#7987,#6131,#6132);
#5271=AXIS2_PLACEMENT_3D('',#7988,#6133,#6134);
#6070=DIRECTION('axis',(0.,0.,1.));
#6071=DIRECTION('refdir',(1.,0.,0.));
#6072=DIRECTION('center_axis',(0.,-1.,0.));
#6073=DIRECTION('ref_axis',(1.,0.,0.));
#6074=DIRECTION('center_axis',(0.,-1.,0.));
#6075=DIRECTION('ref_axis',(1.,0.,0.));
#6076=DIRECTION('',(0.,1.,0.));
#6077=DIRECTION('center_axis',(0.,-1.,0.));
#6078=DIRECTION('ref_axis',(1.,0.,0.));
#6079=DIRECTION('center_axis',(0.,1.,0.));
#6080=DIRECTION('ref_axis',(0.,0.,1.));
#6081=DIRECTION('center_axis',(0.,-1.,0.));
#6082=DIRECTION('ref_axis',(1.,0.,0.));
#6083=DIRECTION('center_axis',(6.12323399573677E-17,0.,1.));
#6084=DIRECTION('ref_axis',(1.,0.,0.));
#6085=DIRECTION('center_axis',(1.22464679914735E-16,-1.,0.));
#6086=DIRECTION('ref_axis',(-1.,-1.22464679914735E-16,0.));
#6087=DIRECTION('center_axis',(0.,-1.,0.));
#6088=DIRECTION('ref_axis',(1.,0.,0.));
#6089=DIRECTION('center_axis',(0.,-1.,0.));
#6090=DIRECTION('ref_axis',(0.,0.,-1.));
#6091=DIRECTION('center_axis',(-0.866025403784438,0.,-0.5));
#6092=DIRECTION('ref_axis',(-0.5,0.,0.866025403784438));
#6093=DIRECTION('',(-0.866025403784438,0.,-0.5));
#6094=DIRECTION('center_axis',(-0.866025403784438,0.,-0.5));
#6095=DIRECTION('ref_axis',(-0.5,0.,0.866025403784438));
#6096=DIRECTION('',(-0.866025403784438,0.,-0.5));
#6097=DIRECTION('center_axis',(0.,-1.,0.));
#6098=DIRECTION('ref_axis',(1.,0.,0.));
#6099=DIRECTION('center_axis',(0.,-1.,0.));
#6100=DIRECTION('ref_axis',(1.,0.,0.));
#6101=DIRECTION('',(0.,1.,0.));
#6102=DIRECTION('center_axis',(0.,-1.,0.));
#6103=DIRECTION('ref_axis',(1.,0.,0.));
#6104=DIRECTION('center_axis',(0.866025403784439,0.,-0.5));
#6105=DIRECTION('ref_axis',(-0.5,0.,-0.866025403784439));
#6106=DIRECTION('',(0.866025403784439,0.,-0.5));
#6107=DIRECTION('center_axis',(0.866025403784439,0.,-0.5));
#6108=DIRECTION('ref_axis',(-0.5,0.,-0.866025403784439));
#6109=DIRECTION('',(0.866025403784439,0.,-0.5));
#6110=DIRECTION('center_axis',(0.,0.,1.));
#6111=DIRECTION('ref_axis',(1.,0.,0.));
#6112=DIRECTION('',(0.,0.,1.));
#6113=DIRECTION('center_axis',(0.,0.,1.));
#6114=DIRECTION('ref_axis',(1.,0.,0.));
#6115=DIRECTION('',(0.,0.,1.));
#6116=DIRECTION('center_axis',(0.,1.,0.));
#6117=DIRECTION('ref_axis',(0.,0.,1.));
#6118=DIRECTION('center_axis',(0.,-1.,0.));
#6119=DIRECTION('ref_axis',(1.,0.,0.));
#6120=DIRECTION('center_axis',(0.,1.,0.));
#6121=DIRECTION('ref_axis',(0.,0.,1.));
#6122=DIRECTION('center_axis',(0.,-1.,0.));
#6123=DIRECTION('ref_axis',(1.,0.,0.));
#6124=DIRECTION('center_axis',(0.,-1.,0.));
#6125=DIRECTION('ref_axis',(1.,0.,0.));
#6126=DIRECTION('center_axis',(0.,-1.,0.));
#6127=DIRECTION('ref_axis',(1.,0.,0.));
#6128=DIRECTION('',(0.,1.,0.));
#6129=DIRECTION('center_axis',(0.,-1.,0.));
#6130=DIRECTION('ref_axis',(0.,0.,-1.));
#6131=DIRECTION('center_axis',(0.,-1.,0.));
#6132=DIRECTION('ref_axis',(1.,0.,0.));
#6133=DIRECTION('center_axis',(0.,-1.,0.));
#6134=DIRECTION('ref_axis',(1.,0.,0.));
#6135=DIRECTION('',(0.,1.,0.));
#7484=CARTESIAN_POINT('',(0.,0.,0.));
#7485=CARTESIAN_POINT('Origin',(0.,0.,0.));
#7486=CARTESIAN_POINT('',(-1.8,-0.85,-2.20436423846524E-16));
#7487=CARTESIAN_POINT('Origin',(0.,-0.85,0.));
#7488=CARTESIAN_POINT('',(-1.8,0.85,-2.20436423846524E-16));
#7489=CARTESIAN_POINT('',(-1.8,0.,-2.20436423846524E-16));
#7490=CARTESIAN_POINT('Origin',(0.,0.85,0.));
#7491=CARTESIAN_POINT('Origin',(2.19089023002066,0.85,0.));
#7492=CARTESIAN_POINT('',(2.19089023002066,0.85,0.));
#7493=CARTESIAN_POINT('Origin',(0.,0.85,0.));
#7494=CARTESIAN_POINT('Origin',(3.99680288865056E-15,0.,0.));
#7495=CARTESIAN_POINT('',(3.85290688975075E-15,-1.76221774462768E-32,2.35));
#7496=CARTESIAN_POINT('',(3.85290688975075E-15,-1.76221774462768E-32,-2.35));
#7497=CARTESIAN_POINT('Origin',(3.99680288865056E-15,0.,0.));
#7498=CARTESIAN_POINT('',(2.19089023002066,-0.85,0.));
#7499=CARTESIAN_POINT('Origin',(0.,-0.85,0.));
#7500=CARTESIAN_POINT('Origin',(1.8,-0.85,0.));
#7501=CARTESIAN_POINT('Origin',(0.,1.55,0.));
#7502=CARTESIAN_POINT('',(1.42894191624432,1.8,0.825000000000001));
#7503=CARTESIAN_POINT('',(1.53744468918255,1.55,0.598968970568896));
#7504=CARTESIAN_POINT('Ctrl Pts',(1.42894191624432,1.8,0.825000000000001));
#7505=CARTESIAN_POINT('Ctrl Pts',(1.44466308895875,1.8,0.797770130104052));
#7506=CARTESIAN_POINT('Ctrl Pts',(1.46055812562105,1.79370633789704,0.768258557763732));
#7507=CARTESIAN_POINT('Ctrl Pts',(1.48824888379079,1.76817777258318,0.713138492740816));
#7508=CARTESIAN_POINT('Ctrl Pts',(1.50008999307766,1.74894552961493,0.687551581002689));
#7509=CARTESIAN_POINT('Ctrl Pts',(1.51812136280714,1.70460745840382,0.646764802471699));
#7510=CARTESIAN_POINT('Ctrl Pts',(1.52552758004446,1.67652816181843,0.628833667319578));
#7511=CARTESIAN_POINT('Ctrl Pts',(1.53516661651472,1.61494799959182,0.604921184808251));
#7512=CARTESIAN_POINT('Ctrl Pts',(1.53744468918255,1.58144291640553,0.598968970568896));
#7513=CARTESIAN_POINT('Ctrl Pts',(1.53744468918255,1.55,0.598968970568896));
#7514=CARTESIAN_POINT('',(1.42894191624432,1.3,0.825000000000001));
#7515=CARTESIAN_POINT('Ctrl Pts',(1.42894191624432,1.3,0.825000000000001));
#7516=CARTESIAN_POINT('Ctrl Pts',(1.4132207435299,1.3,0.852229869895949));
#7517=CARTESIAN_POINT('Ctrl Pts',(1.39561049050871,1.30629366210296,0.880751161609749));
#7518=CARTESIAN_POINT('Ctrl Pts',(1.36172049302549,1.33182222741682,0.932292094146256));
#7519=CARTESIAN_POINT('Ctrl Pts',(1.34548213209931,1.35105447038507,0.955340251466734));
#7520=CARTESIAN_POINT('Ctrl Pts',(1.31917543061769,1.39539254159618,0.99134926498299));
#7521=CARTESIAN_POINT('Ctrl Pts',(1.30734972067592,1.42347183818157,1.00672880483252));
#7522=CARTESIAN_POINT('Ctrl Pts',(1.29146042158868,1.48505200040818,1.02703269653942));
#7523=CARTESIAN_POINT('Ctrl Pts',(1.28744468918255,1.51855708359447,1.03198167246111));
#7524=CARTESIAN_POINT('Ctrl Pts',(1.28744468918255,1.58144291640553,1.03198167246111));
#7525=CARTESIAN_POINT('Ctrl Pts',(1.29146042158868,1.61494799959182,1.02703269653942));
#7526=CARTESIAN_POINT('Ctrl Pts',(1.30734972067592,1.67652816181843,1.00672880483252));
#7527=CARTESIAN_POINT('Ctrl Pts',(1.31917543061769,1.70460745840382,0.991349264982991));
#7528=CARTESIAN_POINT('Ctrl Pts',(1.34548213209931,1.74894552961493,0.955340251466735));
#7529=CARTESIAN_POINT('Ctrl Pts',(1.36172049302549,1.76817777258318,0.932292094146256));
#7530=CARTESIAN_POINT('Ctrl Pts',(1.39561049050871,1.79370633789704,0.880751161609749));
#7531=CARTESIAN_POINT('Ctrl Pts',(1.4132207435299,1.8,0.85222986989595));
#7532=CARTESIAN_POINT('Ctrl Pts',(1.42894191624432,1.8,0.825000000000001));
#7533=CARTESIAN_POINT('Ctrl Pts',(1.53744468918255,1.55,0.598968970568896));
#7534=CARTESIAN_POINT('Ctrl Pts',(1.53744468918255,1.51855708359447,0.598968970568896));
#7535=CARTESIAN_POINT('Ctrl Pts',(1.53516661651472,1.48505200040818,0.60492118480825));
#7536=CARTESIAN_POINT('Ctrl Pts',(1.52552758004446,1.42347183818157,0.628833667319578));
#7537=CARTESIAN_POINT('Ctrl Pts',(1.51812136280714,1.39539254159618,0.646764802471699));
#7538=CARTESIAN_POINT('Ctrl Pts',(1.50008999307766,1.35105447038507,0.687551581002689));
#7539=CARTESIAN_POINT('Ctrl Pts',(1.48824888379079,1.33182222741682,0.713138492740816));
#7540=CARTESIAN_POINT('Ctrl Pts',(1.46055812562105,1.30629366210296,0.768258557763732));
#7541=CARTESIAN_POINT('Ctrl Pts',(1.44466308895875,1.3,0.797770130104052));
#7542=CARTESIAN_POINT('Ctrl Pts',(1.42894191624432,1.3,0.825000000000001));
#7543=CARTESIAN_POINT('',(0.963525491562421,1.55,0.267616567329818));
#7544=CARTESIAN_POINT('',(0.125,1.55,-0.21650635094611));
#7545=CARTESIAN_POINT('Ctrl Pts',(0.963525491562421,1.55,0.267616567329818));
#7546=CARTESIAN_POINT('Ctrl Pts',(0.963525491562421,1.5815373526696,0.267616567329818));
#7547=CARTESIAN_POINT('Ctrl Pts',(0.961833761492987,1.61508042700263,0.273949373987484));
#7548=CARTESIAN_POINT('Ctrl Pts',(0.954308486908894,1.67663267125761,0.299111603474268));
#7549=CARTESIAN_POINT('Ctrl Pts',(0.948394987258249,1.70465411363682,0.31788699900678));
#7550=CARTESIAN_POINT('Ctrl Pts',(0.933155485613026,1.74889618382539,0.360174810895352));
#7551=CARTESIAN_POINT('Ctrl Pts',(0.92278792026947,1.76811531482682,0.386546956384144));
#7552=CARTESIAN_POINT('Ctrl Pts',(0.897143218189782,1.79367084275751,0.442820664919227));
#7553=CARTESIAN_POINT('Ctrl Pts',(0.881791875377343,1.8,0.472691670144998));
#7554=CARTESIAN_POINT('Ctrl Pts',(0.850258932191534,1.8,0.527308329855003));
#7555=CARTESIAN_POINT('Ctrl Pts',(0.832065554235658,1.79367084275751,0.555538485325664));
#7556=CARTESIAN_POINT('Ctrl Pts',(0.796153444118959,1.76811531482682,0.605884303066698));
#7557=CARTESIAN_POINT('Ctrl Pts',(0.778498278845144,1.74889618382539,0.62804895077401));
#7558=CARTESIAN_POINT('Ctrl Pts',(0.749495710301794,1.70465411363682,0.662390652284073));
#7559=CARTESIAN_POINT('Ctrl Pts',(0.73619249062986,1.67663267125761,0.676899590973058));
#7560=CARTESIAN_POINT('Ctrl Pts',(0.718163997970498,1.61508042700263,0.695997784676728));
#7561=CARTESIAN_POINT('Ctrl Pts',(0.713525491562421,1.5815373526696,0.700629269222037));
#7562=CARTESIAN_POINT('Ctrl Pts',(0.713525491562421,1.5184626473304,0.700629269222037));
#7563=CARTESIAN_POINT('Ctrl Pts',(0.718163997970498,1.48491957299737,0.695997784676728));
#7564=CARTESIAN_POINT('Ctrl Pts',(0.73619249062986,1.42336732874239,0.676899590973058));
#7565=CARTESIAN_POINT('Ctrl Pts',(0.749495710301794,1.39534588636318,0.662390652284073));
#7566=CARTESIAN_POINT('Ctrl Pts',(0.778498278845144,1.35110381617461,0.62804895077401));
#7567=CARTESIAN_POINT('Ctrl Pts',(0.796153444118959,1.33188468517318,0.605884303066698));
#7568=CARTESIAN_POINT('Ctrl Pts',(0.832065554235658,1.30632915724249,0.555538485325664));
#7569=CARTESIAN_POINT('Ctrl Pts',(0.850258932191534,1.3,0.527308329855003));
#7570=CARTESIAN_POINT('Ctrl Pts',(0.881791875377343,1.3,0.472691670144998));
#7571=CARTESIAN_POINT('Ctrl Pts',(0.897143218189782,1.30632915724249,0.442820664919227));
#7572=CARTESIAN_POINT('Ctrl Pts',(0.92278792026947,1.33188468517318,0.386546956384144));
#7573=CARTESIAN_POINT('Ctrl Pts',(0.933155485613026,1.35110381617461,0.360174810895352));
#7574=CARTESIAN_POINT('Ctrl Pts',(0.948394987258249,1.39534588636318,0.31788699900678));
#7575=CARTESIAN_POINT('Ctrl Pts',(0.954308486908894,1.42336732874239,0.299111603474268));
#7576=CARTESIAN_POINT('Ctrl Pts',(0.961833761492987,1.48491957299738,0.273949373987484));
#7577=CARTESIAN_POINT('Ctrl Pts',(0.963525491562421,1.5184626473304,0.267616567329818));
#7578=CARTESIAN_POINT('Ctrl Pts',(0.963525491562421,1.55,0.267616567329818));
#7579=CARTESIAN_POINT('Origin',(0.,1.55,0.));
#7580=CARTESIAN_POINT('',(-0.713525491562421,1.55,-0.700629269222037));
#7581=CARTESIAN_POINT('Ctrl Pts',(-0.713525491562421,1.55,-0.700629269222037));
#7582=CARTESIAN_POINT('Ctrl Pts',(-0.713525491562421,1.5184626473304,-0.700629269222037));
#7583=CARTESIAN_POINT('Ctrl Pts',(-0.718163997970498,1.48491957299737,-0.695997784676728));
#7584=CARTESIAN_POINT('Ctrl Pts',(-0.73619249062986,1.42336732874239,-0.676899590973058));
#7585=CARTESIAN_POINT('Ctrl Pts',(-0.749495710301794,1.39534588636318,-0.662390652284073));
#7586=CARTESIAN_POINT('Ctrl Pts',(-0.778498278845144,1.35110381617461,-0.62804895077401));
#7587=CARTESIAN_POINT('Ctrl Pts',(-0.796153444118959,1.33188468517318,-0.605884303066698));
#7588=CARTESIAN_POINT('Ctrl Pts',(-0.832065554235658,1.30632915724249,-0.555538485325664));
#7589=CARTESIAN_POINT('Ctrl Pts',(-0.850258932191534,1.3,-0.527308329855003));
#7590=CARTESIAN_POINT('Ctrl Pts',(-0.881791875377343,1.3,-0.472691670144998));
#7591=CARTESIAN_POINT('Ctrl Pts',(-0.897143218189782,1.30632915724249,-0.442820664919227));
#7592=CARTESIAN_POINT('Ctrl Pts',(-0.92278792026947,1.33188468517318,-0.386546956384144));
#7593=CARTESIAN_POINT('Ctrl Pts',(-0.933155485613026,1.35110381617461,-0.360174810895352));
#7594=CARTESIAN_POINT('Ctrl Pts',(-0.948394987258249,1.39534588636318,-0.31788699900678));
#7595=CARTESIAN_POINT('Ctrl Pts',(-0.954308486908894,1.42336732874239,-0.299111603474268));
#7596=CARTESIAN_POINT('Ctrl Pts',(-0.961833761492986,1.48491957299737,-0.273949373987484));
#7597=CARTESIAN_POINT('Ctrl Pts',(-0.963525491562421,1.5184626473304,-0.267616567329818));
#7598=CARTESIAN_POINT('Ctrl Pts',(-0.963525491562421,1.5815373526696,-0.267616567329818));
#7599=CARTESIAN_POINT('Ctrl Pts',(-0.961833761492986,1.61508042700263,-0.273949373987484));
#7600=CARTESIAN_POINT('Ctrl Pts',(-0.954308486908894,1.67663267125761,-0.299111603474268));
#7601=CARTESIAN_POINT('Ctrl Pts',(-0.948394987258249,1.70465411363682,-0.31788699900678));
#7602=CARTESIAN_POINT('Ctrl Pts',(-0.933155485613026,1.74889618382539,-0.360174810895352));
#7603=CARTESIAN_POINT('Ctrl Pts',(-0.92278792026947,1.76811531482682,-0.386546956384144));
#7604=CARTESIAN_POINT('Ctrl Pts',(-0.897143218189782,1.79367084275751,-0.442820664919227));
#7605=CARTESIAN_POINT('Ctrl Pts',(-0.881791875377343,1.8,-0.472691670144998));
#7606=CARTESIAN_POINT('Ctrl Pts',(-0.850258932191534,1.8,-0.527308329855003));
#7607=CARTESIAN_POINT('Ctrl Pts',(-0.832065554235658,1.79367084275751,-0.555538485325664));
#7608=CARTESIAN_POINT('Ctrl Pts',(-0.796153444118959,1.76811531482682,-0.605884303066698));
#7609=CARTESIAN_POINT('Ctrl Pts',(-0.778498278845144,1.74889618382539,-0.62804895077401));
#7610=CARTESIAN_POINT('Ctrl Pts',(-0.749495710301794,1.70465411363682,-0.662390652284073));
#7611=CARTESIAN_POINT('Ctrl Pts',(-0.73619249062986,1.67663267125761,-0.676899590973058));
#7612=CARTESIAN_POINT('Ctrl Pts',(-0.718163997970498,1.61508042700263,-0.695997784676728));
#7613=CARTESIAN_POINT('Ctrl Pts',(-0.713525491562421,1.5815373526696,-0.700629269222037));
#7614=CARTESIAN_POINT('Ctrl Pts',(-0.713525491562421,1.55,-0.700629269222037));
#7615=CARTESIAN_POINT('',(-1.28744468918255,1.55,-1.03198167246111));
#7616=CARTESIAN_POINT('',(0.125,1.55,-0.21650635094611));
#7617=CARTESIAN_POINT('',(-1.42894191624432,1.3,-0.825000000000001));
#7618=CARTESIAN_POINT('Ctrl Pts',(-1.42894191624432,1.3,-0.825000000000001));
#7619=CARTESIAN_POINT('Ctrl Pts',(-1.4132207435299,1.3,-0.852229869895949));
#7620=CARTESIAN_POINT('Ctrl Pts',(-1.39561049050871,1.30629366210296,-0.880751161609749));
#7621=CARTESIAN_POINT('Ctrl Pts',(-1.36172049302549,1.33182222741682,-0.932292094146256));
#7622=CARTESIAN_POINT('Ctrl Pts',(-1.34548213209931,1.35105447038507,-0.955340251466735));
#7623=CARTESIAN_POINT('Ctrl Pts',(-1.31917543061769,1.39539254159618,-0.991349264982991));
#7624=CARTESIAN_POINT('Ctrl Pts',(-1.30734972067592,1.42347183818157,-1.00672880483252));
#7625=CARTESIAN_POINT('Ctrl Pts',(-1.29146042158868,1.48505200040818,-1.02703269653942));
#7626=CARTESIAN_POINT('Ctrl Pts',(-1.28744468918255,1.51855708359447,-1.03198167246111));
#7627=CARTESIAN_POINT('Ctrl Pts',(-1.28744468918255,1.55,-1.03198167246111));
#7628=CARTESIAN_POINT('',(-1.42894191624432,1.8,-0.825000000000001));
#7629=CARTESIAN_POINT('Ctrl Pts',(-1.42894191624432,1.8,-0.825000000000001));
#7630=CARTESIAN_POINT('Ctrl Pts',(-1.44466308895875,1.8,-0.797770130104052));
#7631=CARTESIAN_POINT('Ctrl Pts',(-1.46055812562105,1.79370633789704,-0.768258557763732));
#7632=CARTESIAN_POINT('Ctrl Pts',(-1.48824888379079,1.76817777258318,-0.713138492740816));
#7633=CARTESIAN_POINT('Ctrl Pts',(-1.50008999307766,1.74894552961493,-0.687551581002689));
#7634=CARTESIAN_POINT('Ctrl Pts',(-1.51812136280714,1.70460745840382,-0.646764802471699));
#7635=CARTESIAN_POINT('Ctrl Pts',(-1.52552758004446,1.67652816181843,-0.628833667319578));
#7636=CARTESIAN_POINT('Ctrl Pts',(-1.53516661651472,1.61494799959182,-0.60492118480825));
#7637=CARTESIAN_POINT('Ctrl Pts',(-1.53744468918255,1.58144291640553,-0.598968970568896));
#7638=CARTESIAN_POINT('Ctrl Pts',(-1.53744468918255,1.51855708359447,-0.598968970568896));
#7639=CARTESIAN_POINT('Ctrl Pts',(-1.53516661651472,1.48505200040818,-0.60492118480825));
#7640=CARTESIAN_POINT('Ctrl Pts',(-1.52552758004446,1.42347183818157,-0.628833667319578));
#7641=CARTESIAN_POINT('Ctrl Pts',(-1.51812136280714,1.39539254159618,-0.646764802471699));
#7642=CARTESIAN_POINT('Ctrl Pts',(-1.50008999307766,1.35105447038507,-0.687551581002689));
#7643=CARTESIAN_POINT('Ctrl Pts',(-1.48824888379079,1.33182222741682,-0.713138492740816));
#7644=CARTESIAN_POINT('Ctrl Pts',(-1.46055812562105,1.30629366210296,-0.768258557763732));
#7645=CARTESIAN_POINT('Ctrl Pts',(-1.44466308895875,1.3,-0.797770130104052));
#7646=CARTESIAN_POINT('Ctrl Pts',(-1.42894191624432,1.3,-0.825000000000001));
#7647=CARTESIAN_POINT('Ctrl Pts',(-1.28744468918255,1.55,-1.03198167246111));
#7648=CARTESIAN_POINT('Ctrl Pts',(-1.28744468918255,1.58144291640553,-1.03198167246111));
#7649=CARTESIAN_POINT('Ctrl Pts',(-1.29146042158868,1.61494799959182,-1.02703269653942));
#7650=CARTESIAN_POINT('Ctrl Pts',(-1.30734972067592,1.67652816181843,-1.00672880483252));
#7651=CARTESIAN_POINT('Ctrl Pts',(-1.31917543061769,1.70460745840382,-0.991349264982991));
#7652=CARTESIAN_POINT('Ctrl Pts',(-1.34548213209931,1.74894552961493,-0.955340251466734));
#7653=CARTESIAN_POINT('Ctrl Pts',(-1.36172049302549,1.76817777258318,-0.932292094146256));
#7654=CARTESIAN_POINT('Ctrl Pts',(-1.39561049050871,1.79370633789704,-0.880751161609749));
#7655=CARTESIAN_POINT('Ctrl Pts',(-1.4132207435299,1.8,-0.852229869895949));
#7656=CARTESIAN_POINT('Ctrl Pts',(-1.42894191624432,1.8,-0.825000000000001));
#7657=CARTESIAN_POINT('Origin',(0.,1.55,0.));
#7658=CARTESIAN_POINT('',(-1.65,0.85,-2.02066721859313E-16));
#7659=CARTESIAN_POINT('Origin',(0.,0.85,0.));
#7660=CARTESIAN_POINT('',(-1.65,2.25,-2.02066721859313E-16));
#7661=CARTESIAN_POINT('',(-1.65,1.55,-2.02066721859313E-16));
#7662=CARTESIAN_POINT('Origin',(0.,2.25,0.));
#7663=CARTESIAN_POINT('',(-1.42894191624432,1.3,0.825));
#7664=CARTESIAN_POINT('',(-1.42894191624432,1.8,0.825));
#7665=CARTESIAN_POINT('Ctrl Pts',(-1.42894191624432,1.3,0.825));
#7666=CARTESIAN_POINT('Ctrl Pts',(-1.44466308895875,1.3,0.797770130104051));
#7667=CARTESIAN_POINT('Ctrl Pts',(-1.46055812562105,1.30629366210296,0.768258557763731));
#7668=CARTESIAN_POINT('Ctrl Pts',(-1.48824888379079,1.33182222741682,0.713138492740815));
#7669=CARTESIAN_POINT('Ctrl Pts',(-1.50008999307766,1.35105447038507,0.687551581002688));
#7670=CARTESIAN_POINT('Ctrl Pts',(-1.51812136280714,1.39539254159618,0.646764802471698));
#7671=CARTESIAN_POINT('Ctrl Pts',(-1.52552758004446,1.42347183818157,0.628833667319577));
#7672=CARTESIAN_POINT('Ctrl Pts',(-1.53516661651472,1.48505200040818,0.604921184808249));
#7673=CARTESIAN_POINT('Ctrl Pts',(-1.53744468918255,1.51855708359447,0.598968970568895));
#7674=CARTESIAN_POINT('Ctrl Pts',(-1.53744468918255,1.58144291640553,0.598968970568895));
#7675=CARTESIAN_POINT('Ctrl Pts',(-1.53516661651472,1.61494799959182,0.604921184808249));
#7676=CARTESIAN_POINT('Ctrl Pts',(-1.52552758004446,1.67652816181843,0.628833667319577));
#7677=CARTESIAN_POINT('Ctrl Pts',(-1.51812136280714,1.70460745840382,0.646764802471698));
#7678=CARTESIAN_POINT('Ctrl Pts',(-1.50008999307766,1.74894552961493,0.687551581002688));
#7679=CARTESIAN_POINT('Ctrl Pts',(-1.48824888379079,1.76817777258318,0.713138492740815));
#7680=CARTESIAN_POINT('Ctrl Pts',(-1.46055812562105,1.79370633789704,0.768258557763731));
#7681=CARTESIAN_POINT('Ctrl Pts',(-1.44466308895875,1.8,0.797770130104051));
#7682=CARTESIAN_POINT('Ctrl Pts',(-1.42894191624432,1.8,0.825));
#7683=CARTESIAN_POINT('',(-1.28744468918255,1.55,1.03198167246111));
#7684=CARTESIAN_POINT('Ctrl Pts',(-1.42894191624432,1.8,0.825));
#7685=CARTESIAN_POINT('Ctrl Pts',(-1.4132207435299,1.8,0.852229869895948));
#7686=CARTESIAN_POINT('Ctrl Pts',(-1.39561049050871,1.79370633789704,0.880751161609747));
#7687=CARTESIAN_POINT('Ctrl Pts',(-1.36172049302549,1.76817777258318,0.932292094146255));
#7688=CARTESIAN_POINT('Ctrl Pts',(-1.34548213209931,1.74894552961493,0.955340251466733));
#7689=CARTESIAN_POINT('Ctrl Pts',(-1.31917543061769,1.70460745840382,0.991349264982989));
#7690=CARTESIAN_POINT('Ctrl Pts',(-1.30734972067592,1.67652816181843,1.00672880483252));
#7691=CARTESIAN_POINT('Ctrl Pts',(-1.29146042158868,1.61494799959182,1.02703269653942));
#7692=CARTESIAN_POINT('Ctrl Pts',(-1.28744468918255,1.58144291640553,1.03198167246111));
#7693=CARTESIAN_POINT('Ctrl Pts',(-1.28744468918255,1.55,1.03198167246111));
#7694=CARTESIAN_POINT('Ctrl Pts',(-1.28744468918255,1.55,1.03198167246111));
#7695=CARTESIAN_POINT('Ctrl Pts',(-1.28744468918255,1.51855708359447,1.03198167246111));
#7696=CARTESIAN_POINT('Ctrl Pts',(-1.29146042158868,1.48505200040818,1.02703269653942));
#7697=CARTESIAN_POINT('Ctrl Pts',(-1.30734972067592,1.42347183818157,1.00672880483252));
#7698=CARTESIAN_POINT('Ctrl Pts',(-1.31917543061769,1.39539254159618,0.99134926498299));
#7699=CARTESIAN_POINT('Ctrl Pts',(-1.34548213209931,1.35105447038508,0.955340251466733));
#7700=CARTESIAN_POINT('Ctrl Pts',(-1.36172049302549,1.33182222741682,0.932292094146255));
#7701=CARTESIAN_POINT('Ctrl Pts',(-1.39561049050871,1.30629366210296,0.880751161609748));
#7702=CARTESIAN_POINT('Ctrl Pts',(-1.4132207435299,1.3,0.852229869895949));
#7703=CARTESIAN_POINT('Ctrl Pts',(-1.42894191624432,1.3,0.825));
#7704=CARTESIAN_POINT('',(1.42894191624432,1.8,-0.825));
#7705=CARTESIAN_POINT('',(1.42894191624432,1.3,-0.825));
#7706=CARTESIAN_POINT('Ctrl Pts',(1.42894191624432,1.8,-0.825));
#7707=CARTESIAN_POINT('Ctrl Pts',(1.4132207435299,1.8,-0.852229869895949));
#7708=CARTESIAN_POINT('Ctrl Pts',(1.39561049050871,1.79370633789704,-0.880751161609748));
#7709=CARTESIAN_POINT('Ctrl Pts',(1.36172049302549,1.76817777258318,-0.932292094146255));
#7710=CARTESIAN_POINT('Ctrl Pts',(1.34548213209931,1.74894552961493,-0.955340251466734));
#7711=CARTESIAN_POINT('Ctrl Pts',(1.31917543061769,1.70460745840382,-0.99134926498299));
#7712=CARTESIAN_POINT('Ctrl Pts',(1.30734972067592,1.67652816181843,-1.00672880483252));
#7713=CARTESIAN_POINT('Ctrl Pts',(1.29146042158868,1.61494799959182,-1.02703269653942));
#7714=CARTESIAN_POINT('Ctrl Pts',(1.28744468918255,1.58144291640553,-1.03198167246111));
#7715=CARTESIAN_POINT('Ctrl Pts',(1.28744468918255,1.51855708359447,-1.03198167246111));
#7716=CARTESIAN_POINT('Ctrl Pts',(1.29146042158868,1.48505200040818,-1.02703269653942));
#7717=CARTESIAN_POINT('Ctrl Pts',(1.30734972067592,1.42347183818157,-1.00672880483252));
#7718=CARTESIAN_POINT('Ctrl Pts',(1.31917543061769,1.39539254159618,-0.99134926498299));
#7719=CARTESIAN_POINT('Ctrl Pts',(1.34548213209931,1.35105447038507,-0.955340251466734));
#7720=CARTESIAN_POINT('Ctrl Pts',(1.36172049302549,1.33182222741682,-0.932292094146255));
#7721=CARTESIAN_POINT('Ctrl Pts',(1.39561049050871,1.30629366210296,-0.880751161609748));
#7722=CARTESIAN_POINT('Ctrl Pts',(1.4132207435299,1.3,-0.852229869895948));
#7723=CARTESIAN_POINT('Ctrl Pts',(1.42894191624432,1.3,-0.825));
#7724=CARTESIAN_POINT('',(1.53744468918255,1.55,-0.598968970568895));
#7725=CARTESIAN_POINT('Ctrl Pts',(1.42894191624432,1.3,-0.825));
#7726=CARTESIAN_POINT('Ctrl Pts',(1.44466308895875,1.3,-0.797770130104051));
#7727=CARTESIAN_POINT('Ctrl Pts',(1.46055812562105,1.30629366210296,-0.768258557763731));
#7728=CARTESIAN_POINT('Ctrl Pts',(1.48824888379079,1.33182222741682,-0.713138492740815));
#7729=CARTESIAN_POINT('Ctrl Pts',(1.50008999307766,1.35105447038507,-0.687551581002688));
#7730=CARTESIAN_POINT('Ctrl Pts',(1.51812136280714,1.39539254159618,-0.646764802471698));
#7731=CARTESIAN_POINT('Ctrl Pts',(1.52552758004446,1.42347183818157,-0.628833667319577));
#7732=CARTESIAN_POINT('Ctrl Pts',(1.53516661651472,1.48505200040818,-0.604921184808249));
#7733=CARTESIAN_POINT('Ctrl Pts',(1.53744468918255,1.51855708359447,-0.598968970568895));
#7734=CARTESIAN_POINT('Ctrl Pts',(1.53744468918255,1.55,-0.598968970568895));
#7735=CARTESIAN_POINT('Ctrl Pts',(1.53744468918255,1.55,-0.598968970568895));
#7736=CARTESIAN_POINT('Ctrl Pts',(1.53744468918255,1.58144291640553,-0.598968970568895));
#7737=CARTESIAN_POINT('Ctrl Pts',(1.53516661651472,1.61494799959182,-0.604921184808249));
#7738=CARTESIAN_POINT('Ctrl Pts',(1.52552758004446,1.67652816181843,-0.628833667319577));
#7739=CARTESIAN_POINT('Ctrl Pts',(1.51812136280714,1.70460745840382,-0.646764802471698));
#7740=CARTESIAN_POINT('Ctrl Pts',(1.50008999307766,1.74894552961493,-0.687551581002688));
#7741=CARTESIAN_POINT('Ctrl Pts',(1.48824888379079,1.76817777258318,-0.713138492740815));
#7742=CARTESIAN_POINT('Ctrl Pts',(1.46055812562105,1.79370633789704,-0.768258557763731));
#7743=CARTESIAN_POINT('Ctrl Pts',(1.44466308895875,1.8,-0.797770130104051));
#7744=CARTESIAN_POINT('Ctrl Pts',(1.42894191624432,1.8,-0.825));
#7745=CARTESIAN_POINT('',(0.,1.3,-1.65));
#7746=CARTESIAN_POINT('',(0.,1.8,-1.65));
#7747=CARTESIAN_POINT('Ctrl Pts',(1.38777878078145E-17,1.3,-1.65));
#7748=CARTESIAN_POINT('Ctrl Pts',(0.0314423454288489,1.3,-1.65));
#7749=CARTESIAN_POINT('Ctrl Pts',(0.0649476351123396,1.30629366210296,-1.64900971937348));
#7750=CARTESIAN_POINT('Ctrl Pts',(0.126528390765307,1.33182222741682,-1.64543058688707));
#7751=CARTESIAN_POINT('Ctrl Pts',(0.154607860978348,1.35105447038507,-1.64289183246942));
#7752=CARTESIAN_POINT('Ctrl Pts',(0.198945932189457,1.39539254159618,-1.63811406745469));
#7753=CARTESIAN_POINT('Ctrl Pts',(0.218177859368546,1.42347183818157,-1.63556247215209));
#7754=CARTESIAN_POINT('Ctrl Pts',(0.243706194926033,1.48505200040818,-1.63195388134767));
#7755=CARTESIAN_POINT('Ctrl Pts',(0.25,1.51855708359447,-1.63095064303001));
#7756=CARTESIAN_POINT('Ctrl Pts',(0.25,1.58144291640553,-1.63095064303001));
#7757=CARTESIAN_POINT('Ctrl Pts',(0.243706194926033,1.61494799959182,-1.63195388134767));
#7758=CARTESIAN_POINT('Ctrl Pts',(0.218177859368546,1.67652816181843,-1.63556247215209));
#7759=CARTESIAN_POINT('Ctrl Pts',(0.198945932189457,1.70460745840382,-1.63811406745469));
#7760=CARTESIAN_POINT('Ctrl Pts',(0.154607860978349,1.74894552961493,-1.64289183246942));
#7761=CARTESIAN_POINT('Ctrl Pts',(0.126528390765307,1.76817777258318,-1.64543058688707));
#7762=CARTESIAN_POINT('Ctrl Pts',(0.0649476351123398,1.79370633789704,-1.64900971937348));
#7763=CARTESIAN_POINT('Ctrl Pts',(0.031442345428849,1.8,-1.65));
#7764=CARTESIAN_POINT('Ctrl Pts',(7.63278329429795E-17,1.8,-1.65));
#7765=CARTESIAN_POINT('',(-0.25,1.55,-1.63095064303001));
#7766=CARTESIAN_POINT('Ctrl Pts',(9.0205620750794E-17,1.8,-1.65));
#7767=CARTESIAN_POINT('Ctrl Pts',(-0.0314423454288488,1.8,-1.65));
#7768=CARTESIAN_POINT('Ctrl Pts',(-0.0649476351123396,1.79370633789704,
-1.64900971937348));
#7769=CARTESIAN_POINT('Ctrl Pts',(-0.126528390765307,1.76817777258318,-1.64543058688707));
#7770=CARTESIAN_POINT('Ctrl Pts',(-0.154607860978348,1.74894552961493,-1.64289183246942));
#7771=CARTESIAN_POINT('Ctrl Pts',(-0.198945932189456,1.70460745840382,-1.63811406745469));
#7772=CARTESIAN_POINT('Ctrl Pts',(-0.218177859368546,1.67652816181843,-1.63556247215209));
#7773=CARTESIAN_POINT('Ctrl Pts',(-0.243706194926033,1.61494799959182,-1.63195388134767));
#7774=CARTESIAN_POINT('Ctrl Pts',(-0.25,1.58144291640553,-1.63095064303001));
#7775=CARTESIAN_POINT('Ctrl Pts',(-0.25,1.55,-1.63095064303001));
#7776=CARTESIAN_POINT('Ctrl Pts',(-0.25,1.55,-1.63095064303001));
#7777=CARTESIAN_POINT('Ctrl Pts',(-0.25,1.51855708359447,-1.63095064303001));
#7778=CARTESIAN_POINT('Ctrl Pts',(-0.243706194926033,1.48505200040818,-1.63195388134767));
#7779=CARTESIAN_POINT('Ctrl Pts',(-0.218177859368546,1.42347183818157,-1.63556247215209));
#7780=CARTESIAN_POINT('Ctrl Pts',(-0.198945932189457,1.39539254159618,-1.63811406745469));
#7781=CARTESIAN_POINT('Ctrl Pts',(-0.154607860978349,1.35105447038507,-1.64289183246942));
#7782=CARTESIAN_POINT('Ctrl Pts',(-0.126528390765307,1.33182222741682,-1.64543058688707));
#7783=CARTESIAN_POINT('Ctrl Pts',(-0.0649476351123398,1.30629366210296,
-1.64900971937348));
#7784=CARTESIAN_POINT('Ctrl Pts',(-0.031442345428849,1.3,-1.65));
#7785=CARTESIAN_POINT('Ctrl Pts',(-4.85722573273506E-17,1.3,-1.65));
#7786=CARTESIAN_POINT('',(0.,1.8,1.65));
#7787=CARTESIAN_POINT('',(0.,1.3,1.65));
#7788=CARTESIAN_POINT('Ctrl Pts',(8.32667268468867E-17,1.8,1.65));
#7789=CARTESIAN_POINT('Ctrl Pts',(0.031442345428849,1.8,1.65));
#7790=CARTESIAN_POINT('Ctrl Pts',(0.0649476351123398,1.79370633789704,1.64900971937348));
#7791=CARTESIAN_POINT('Ctrl Pts',(0.126528390765307,1.76817777258318,1.64543058688707));
#7792=CARTESIAN_POINT('Ctrl Pts',(0.154607860978349,1.74894552961493,1.64289183246942));
#7793=CARTESIAN_POINT('Ctrl Pts',(0.198945932189457,1.70460745840382,1.63811406745469));
#7794=CARTESIAN_POINT('Ctrl Pts',(0.218177859368546,1.67652816181843,1.63556247215209));
#7795=CARTESIAN_POINT('Ctrl Pts',(0.243706194926033,1.61494799959182,1.63195388134767));
#7796=CARTESIAN_POINT('Ctrl Pts',(0.25,1.58144291640553,1.63095064303001));
#7797=CARTESIAN_POINT('Ctrl Pts',(0.25,1.51855708359447,1.63095064303001));
#7798=CARTESIAN_POINT('Ctrl Pts',(0.243706194926033,1.48505200040818,1.63195388134767));
#7799=CARTESIAN_POINT('Ctrl Pts',(0.218177859368546,1.42347183818157,1.63556247215209));
#7800=CARTESIAN_POINT('Ctrl Pts',(0.198945932189457,1.39539254159618,1.63811406745469));
#7801=CARTESIAN_POINT('Ctrl Pts',(0.154607860978348,1.35105447038507,1.64289183246942));
#7802=CARTESIAN_POINT('Ctrl Pts',(0.126528390765307,1.33182222741682,1.64543058688707));
#7803=CARTESIAN_POINT('Ctrl Pts',(0.0649476351123397,1.30629366210296,1.64900971937348));
#7804=CARTESIAN_POINT('Ctrl Pts',(0.0314423454288488,1.3,1.65));
#7805=CARTESIAN_POINT('Ctrl Pts',(-1.38777878078145E-17,1.3,1.65));
#7806=CARTESIAN_POINT('',(-0.25,1.55,1.63095064303001));
#7807=CARTESIAN_POINT('Ctrl Pts',(-5.55111512312578E-17,1.3,1.65));
#7808=CARTESIAN_POINT('Ctrl Pts',(-0.031442345428849,1.3,1.65));
#7809=CARTESIAN_POINT('Ctrl Pts',(-0.0649476351123398,1.30629366210296,
1.64900971937348));
#7810=CARTESIAN_POINT('Ctrl Pts',(-0.126528390765307,1.33182222741682,1.64543058688707));
#7811=CARTESIAN_POINT('Ctrl Pts',(-0.154607860978349,1.35105447038507,1.64289183246942));
#7812=CARTESIAN_POINT('Ctrl Pts',(-0.198945932189457,1.39539254159618,1.63811406745469));
#7813=CARTESIAN_POINT('Ctrl Pts',(-0.218177859368546,1.42347183818157,1.63556247215209));
#7814=CARTESIAN_POINT('Ctrl Pts',(-0.243706194926033,1.48505200040818,1.63195388134767));
#7815=CARTESIAN_POINT('Ctrl Pts',(-0.25,1.51855708359447,1.63095064303001));
#7816=CARTESIAN_POINT('Ctrl Pts',(-0.25,1.55,1.63095064303001));
#7817=CARTESIAN_POINT('Ctrl Pts',(-0.25,1.55,1.63095064303001));
#7818=CARTESIAN_POINT('Ctrl Pts',(-0.25,1.58144291640553,1.63095064303001));
#7819=CARTESIAN_POINT('Ctrl Pts',(-0.243706194926033,1.61494799959182,1.63195388134767));
#7820=CARTESIAN_POINT('Ctrl Pts',(-0.218177859368546,1.67652816181843,1.63556247215209));
#7821=CARTESIAN_POINT('Ctrl Pts',(-0.198945932189456,1.70460745840382,1.63811406745469));
#7822=CARTESIAN_POINT('Ctrl Pts',(-0.154607860978348,1.74894552961493,1.64289183246942));
#7823=CARTESIAN_POINT('Ctrl Pts',(-0.126528390765307,1.76817777258318,1.64543058688707));
#7824=CARTESIAN_POINT('Ctrl Pts',(-0.0649476351123396,1.79370633789704,
1.64900971937348));
#7825=CARTESIAN_POINT('Ctrl Pts',(-0.0314423454288488,1.8,1.65));
#7826=CARTESIAN_POINT('Ctrl Pts',(7.63278329429795E-17,1.8,1.65));
#7827=CARTESIAN_POINT('Origin',(0.,1.55,0.));
#7828=CARTESIAN_POINT('',(-0.713525491562421,1.55,0.700629269222037));
#7829=CARTESIAN_POINT('',(0.125,1.55,0.21650635094611));
#7830=CARTESIAN_POINT('Ctrl Pts',(-0.713525491562421,1.55,0.700629269222037));
#7831=CARTESIAN_POINT('Ctrl Pts',(-0.713525491562421,1.5815373526696,0.700629269222037));
#7832=CARTESIAN_POINT('Ctrl Pts',(-0.718163997970498,1.61508042700263,0.695997784676727));
#7833=CARTESIAN_POINT('Ctrl Pts',(-0.73619249062986,1.67663267125761,0.676899590973058));
#7834=CARTESIAN_POINT('Ctrl Pts',(-0.749495710301795,1.70465411363682,0.662390652284073));
#7835=CARTESIAN_POINT('Ctrl Pts',(-0.778498278845144,1.74889618382539,0.628048950774009));
#7836=CARTESIAN_POINT('Ctrl Pts',(-0.796153444118959,1.76811531482682,0.605884303066698));
#7837=CARTESIAN_POINT('Ctrl Pts',(-0.832065554235658,1.79367084275751,0.555538485325663));
#7838=CARTESIAN_POINT('Ctrl Pts',(-0.850258932191534,1.8,0.527308329855002));
#7839=CARTESIAN_POINT('Ctrl Pts',(-0.881791875377343,1.8,0.472691670144998));
#7840=CARTESIAN_POINT('Ctrl Pts',(-0.897143218189782,1.79367084275751,0.442820664919227));
#7841=CARTESIAN_POINT('Ctrl Pts',(-0.92278792026947,1.76811531482682,0.386546956384144));
#7842=CARTESIAN_POINT('Ctrl Pts',(-0.933155485613026,1.74889618382539,0.360174810895352));
#7843=CARTESIAN_POINT('Ctrl Pts',(-0.948394987258249,1.70465411363682,0.31788699900678));
#7844=CARTESIAN_POINT('Ctrl Pts',(-0.954308486908894,1.67663267125761,0.299111603474267));
#7845=CARTESIAN_POINT('Ctrl Pts',(-0.961833761492987,1.61508042700263,0.273949373987484));
#7846=CARTESIAN_POINT('Ctrl Pts',(-0.963525491562421,1.5815373526696,0.267616567329817));
#7847=CARTESIAN_POINT('Ctrl Pts',(-0.963525491562421,1.5184626473304,0.267616567329817));
#7848=CARTESIAN_POINT('Ctrl Pts',(-0.961833761492987,1.48491957299737,0.273949373987484));
#7849=CARTESIAN_POINT('Ctrl Pts',(-0.954308486908894,1.42336732874239,0.299111603474267));
#7850=CARTESIAN_POINT('Ctrl Pts',(-0.948394987258249,1.39534588636318,0.31788699900678));
#7851=CARTESIAN_POINT('Ctrl Pts',(-0.933155485613026,1.35110381617461,0.360174810895352));
#7852=CARTESIAN_POINT('Ctrl Pts',(-0.92278792026947,1.33188468517318,0.386546956384144));
#7853=CARTESIAN_POINT('Ctrl Pts',(-0.897143218189782,1.30632915724249,0.442820664919227));
#7854=CARTESIAN_POINT('Ctrl Pts',(-0.881791875377343,1.3,0.472691670144998));
#7855=CARTESIAN_POINT('Ctrl Pts',(-0.850258932191534,1.3,0.527308329855002));
#7856=CARTESIAN_POINT('Ctrl Pts',(-0.832065554235658,1.30632915724249,0.555538485325663));
#7857=CARTESIAN_POINT('Ctrl Pts',(-0.796153444118959,1.33188468517318,0.605884303066698));
#7858=CARTESIAN_POINT('Ctrl Pts',(-0.778498278845144,1.35110381617461,0.628048950774009));
#7859=CARTESIAN_POINT('Ctrl Pts',(-0.749495710301795,1.39534588636318,0.662390652284073));
#7860=CARTESIAN_POINT('Ctrl Pts',(-0.73619249062986,1.42336732874239,0.676899590973058));
#7861=CARTESIAN_POINT('Ctrl Pts',(-0.718163997970498,1.48491957299737,0.695997784676727));
#7862=CARTESIAN_POINT('Ctrl Pts',(-0.713525491562421,1.5184626473304,0.700629269222037));
#7863=CARTESIAN_POINT('Ctrl Pts',(-0.713525491562421,1.55,0.700629269222037));
#7864=CARTESIAN_POINT('Origin',(0.,1.55,0.));
#7865=CARTESIAN_POINT('',(0.963525491562421,1.55,-0.267616567329817));
#7866=CARTESIAN_POINT('Ctrl Pts',(0.963525491562421,1.55,-0.267616567329817));
#7867=CARTESIAN_POINT('Ctrl Pts',(0.963525491562421,1.5184626473304,-0.267616567329817));
#7868=CARTESIAN_POINT('Ctrl Pts',(0.961833761492987,1.48491957299737,-0.273949373987484));
#7869=CARTESIAN_POINT('Ctrl Pts',(0.954308486908894,1.42336732874239,-0.299111603474267));
#7870=CARTESIAN_POINT('Ctrl Pts',(0.948394987258249,1.39534588636318,-0.31788699900678));
#7871=CARTESIAN_POINT('Ctrl Pts',(0.933155485613026,1.35110381617461,-0.360174810895352));
#7872=CARTESIAN_POINT('Ctrl Pts',(0.92278792026947,1.33188468517318,-0.386546956384144));
#7873=CARTESIAN_POINT('Ctrl Pts',(0.897143218189782,1.30632915724249,-0.442820664919227));
#7874=CARTESIAN_POINT('Ctrl Pts',(0.881791875377343,1.3,-0.472691670144998));
#7875=CARTESIAN_POINT('Ctrl Pts',(0.850258932191534,1.3,-0.527308329855002));
#7876=CARTESIAN_POINT('Ctrl Pts',(0.832065554235658,1.30632915724249,-0.555538485325663));
#7877=CARTESIAN_POINT('Ctrl Pts',(0.796153444118959,1.33188468517318,-0.605884303066698));
#7878=CARTESIAN_POINT('Ctrl Pts',(0.778498278845144,1.35110381617461,-0.628048950774009));
#7879=CARTESIAN_POINT('Ctrl Pts',(0.749495710301795,1.39534588636318,-0.662390652284073));
#7880=CARTESIAN_POINT('Ctrl Pts',(0.73619249062986,1.42336732874239,-0.676899590973058));
#7881=CARTESIAN_POINT('Ctrl Pts',(0.718163997970498,1.48491957299737,-0.695997784676727));
#7882=CARTESIAN_POINT('Ctrl Pts',(0.713525491562421,1.5184626473304,-0.700629269222037));
#7883=CARTESIAN_POINT('Ctrl Pts',(0.713525491562421,1.5815373526696,-0.700629269222037));
#7884=CARTESIAN_POINT('Ctrl Pts',(0.718163997970498,1.61508042700263,-0.695997784676727));
#7885=CARTESIAN_POINT('Ctrl Pts',(0.73619249062986,1.67663267125761,-0.676899590973058));
#7886=CARTESIAN_POINT('Ctrl Pts',(0.749495710301795,1.70465411363682,-0.662390652284073));
#7887=CARTESIAN_POINT('Ctrl Pts',(0.778498278845144,1.74889618382539,-0.628048950774009));
#7888=CARTESIAN_POINT('Ctrl Pts',(0.796153444118959,1.76811531482682,-0.605884303066698));
#7889=CARTESIAN_POINT('Ctrl Pts',(0.832065554235658,1.79367084275751,-0.555538485325663));
#7890=CARTESIAN_POINT('Ctrl Pts',(0.850258932191534,1.8,-0.527308329855002));
#7891=CARTESIAN_POINT('Ctrl Pts',(0.881791875377343,1.8,-0.472691670144998));
#7892=CARTESIAN_POINT('Ctrl Pts',(0.897143218189782,1.79367084275751,-0.442820664919227));
#7893=CARTESIAN_POINT('Ctrl Pts',(0.92278792026947,1.76811531482682,-0.386546956384144));
#7894=CARTESIAN_POINT('Ctrl Pts',(0.933155485613026,1.74889618382539,-0.360174810895352));
#7895=CARTESIAN_POINT('Ctrl Pts',(0.948394987258249,1.70465411363682,-0.31788699900678));
#7896=CARTESIAN_POINT('Ctrl Pts',(0.954308486908894,1.67663267125761,-0.299111603474267));
#7897=CARTESIAN_POINT('Ctrl Pts',(0.961833761492987,1.61508042700263,-0.273949373987484));
#7898=CARTESIAN_POINT('Ctrl Pts',(0.963525491562421,1.5815373526696,-0.267616567329817));
#7899=CARTESIAN_POINT('Ctrl Pts',(0.963525491562421,1.55,-0.267616567329817));
#7900=CARTESIAN_POINT('',(0.125,1.55,0.21650635094611));
#7901=CARTESIAN_POINT('Origin',(0.,1.55,0.));
#7902=CARTESIAN_POINT('',(-0.25,1.55,-0.968245836551854));
#7903=CARTESIAN_POINT('',(-0.25,1.55,0.));
#7904=CARTESIAN_POINT('Ctrl Pts',(-0.25,1.55,-0.968245836551854));
#7905=CARTESIAN_POINT('Ctrl Pts',(-0.25,1.5815373526696,-0.968245836551854));
#7906=CARTESIAN_POINT('Ctrl Pts',(-0.243669763522489,1.61508042700263,-0.969947158664211));
#7907=CARTESIAN_POINT('Ctrl Pts',(-0.218115996279034,1.67663267125761,-0.976011194447325));
#7908=CARTESIAN_POINT('Ctrl Pts',(-0.198899276956455,1.70465411363682,-0.980277651290853));
#7909=CARTESIAN_POINT('Ctrl Pts',(-0.154657206767882,1.74889618382539,-0.988223761669361));
#7910=CARTESIAN_POINT('Ctrl Pts',(-0.126634476150511,1.76811531482682,-0.992431259450842));
#7911=CARTESIAN_POINT('Ctrl Pts',(-0.0650776639541238,1.79367084275751,
-0.99835915024489));
#7912=CARTESIAN_POINT('Ctrl Pts',(-0.0315329431858092,1.8,-1.));
#7913=CARTESIAN_POINT('Ctrl Pts',(0.0315329431858092,1.8,-1.));
#7914=CARTESIAN_POINT('Ctrl Pts',(0.0650776639541238,1.79367084275751,-0.99835915024489));
#7915=CARTESIAN_POINT('Ctrl Pts',(0.126634476150511,1.76811531482682,-0.992431259450842));
#7916=CARTESIAN_POINT('Ctrl Pts',(0.154657206767882,1.74889618382539,-0.988223761669361));
#7917=CARTESIAN_POINT('Ctrl Pts',(0.198899276956455,1.70465411363682,-0.980277651290853));
#7918=CARTESIAN_POINT('Ctrl Pts',(0.218115996279034,1.67663267125761,-0.976011194447325));
#7919=CARTESIAN_POINT('Ctrl Pts',(0.243669763522488,1.61508042700263,-0.969947158664211));
#7920=CARTESIAN_POINT('Ctrl Pts',(0.25,1.5815373526696,-0.968245836551854));
#7921=CARTESIAN_POINT('Ctrl Pts',(0.25,1.5184626473304,-0.968245836551854));
#7922=CARTESIAN_POINT('Ctrl Pts',(0.243669763522488,1.48491957299737,-0.969947158664211));
#7923=CARTESIAN_POINT('Ctrl Pts',(0.218115996279034,1.42336732874239,-0.976011194447325));
#7924=CARTESIAN_POINT('Ctrl Pts',(0.198899276956455,1.39534588636318,-0.980277651290853));
#7925=CARTESIAN_POINT('Ctrl Pts',(0.154657206767882,1.35110381617461,-0.988223761669361));
#7926=CARTESIAN_POINT('Ctrl Pts',(0.126634476150511,1.33188468517318,-0.992431259450842));
#7927=CARTESIAN_POINT('Ctrl Pts',(0.0650776639541239,1.30632915724249,-0.99835915024489));
#7928=CARTESIAN_POINT('Ctrl Pts',(0.0315329431858092,1.3,-1.));
#7929=CARTESIAN_POINT('Ctrl Pts',(-0.0315329431858092,1.3,-1.));
#7930=CARTESIAN_POINT('Ctrl Pts',(-0.0650776639541239,1.30632915724249,
-0.99835915024489));
#7931=CARTESIAN_POINT('Ctrl Pts',(-0.126634476150511,1.33188468517318,-0.992431259450842));
#7932=CARTESIAN_POINT('Ctrl Pts',(-0.154657206767882,1.35110381617461,-0.988223761669361));
#7933=CARTESIAN_POINT('Ctrl Pts',(-0.198899276956455,1.39534588636318,-0.980277651290853));
#7934=CARTESIAN_POINT('Ctrl Pts',(-0.218115996279034,1.42336732874239,-0.976011194447325));
#7935=CARTESIAN_POINT('Ctrl Pts',(-0.243669763522489,1.48491957299737,-0.969947158664211));
#7936=CARTESIAN_POINT('Ctrl Pts',(-0.25,1.5184626473304,-0.968245836551854));
#7937=CARTESIAN_POINT('Ctrl Pts',(-0.25,1.55,-0.968245836551854));
#7938=CARTESIAN_POINT('Origin',(0.,1.55,0.));
#7939=CARTESIAN_POINT('',(-0.25,1.55,0.968245836551854));
#7940=CARTESIAN_POINT('Ctrl Pts',(-0.25,1.55,0.968245836551854));
#7941=CARTESIAN_POINT('Ctrl Pts',(-0.25,1.5184626473304,0.968245836551854));
#7942=CARTESIAN_POINT('Ctrl Pts',(-0.243669763522489,1.48491957299737,0.969947158664211));
#7943=CARTESIAN_POINT('Ctrl Pts',(-0.218115996279034,1.42336732874239,0.976011194447325));
#7944=CARTESIAN_POINT('Ctrl Pts',(-0.198899276956455,1.39534588636318,0.980277651290853));
#7945=CARTESIAN_POINT('Ctrl Pts',(-0.154657206767882,1.35110381617461,0.988223761669361));
#7946=CARTESIAN_POINT('Ctrl Pts',(-0.126634476150511,1.33188468517318,0.992431259450842));
#7947=CARTESIAN_POINT('Ctrl Pts',(-0.065077663954124,1.30632915724249,0.99835915024489));
#7948=CARTESIAN_POINT('Ctrl Pts',(-0.0315329431858092,1.3,1.));
#7949=CARTESIAN_POINT('Ctrl Pts',(0.0315329431858092,1.3,1.));
#7950=CARTESIAN_POINT('Ctrl Pts',(0.065077663954124,1.30632915724249,0.99835915024489));
#7951=CARTESIAN_POINT('Ctrl Pts',(0.126634476150511,1.33188468517318,0.992431259450842));
#7952=CARTESIAN_POINT('Ctrl Pts',(0.154657206767882,1.35110381617461,0.988223761669361));
#7953=CARTESIAN_POINT('Ctrl Pts',(0.198899276956455,1.39534588636318,0.980277651290853));
#7954=CARTESIAN_POINT('Ctrl Pts',(0.218115996279034,1.42336732874239,0.976011194447325));
#7955=CARTESIAN_POINT('Ctrl Pts',(0.243669763522488,1.48491957299737,0.969947158664211));
#7956=CARTESIAN_POINT('Ctrl Pts',(0.25,1.5184626473304,0.968245836551854));
#7957=CARTESIAN_POINT('Ctrl Pts',(0.25,1.5815373526696,0.968245836551854));
#7958=CARTESIAN_POINT('Ctrl Pts',(0.243669763522488,1.61508042700263,0.969947158664211));
#7959=CARTESIAN_POINT('Ctrl Pts',(0.218115996279034,1.67663267125761,0.976011194447325));
#7960=CARTESIAN_POINT('Ctrl Pts',(0.198899276956455,1.70465411363682,0.980277651290853));
#7961=CARTESIAN_POINT('Ctrl Pts',(0.154657206767882,1.74889618382539,0.988223761669361));
#7962=CARTESIAN_POINT('Ctrl Pts',(0.126634476150511,1.76811531482682,0.992431259450842));
#7963=CARTESIAN_POINT('Ctrl Pts',(0.0650776639541239,1.79367084275751,0.99835915024489));
#7964=CARTESIAN_POINT('Ctrl Pts',(0.0315329431858092,1.8,1.));
#7965=CARTESIAN_POINT('Ctrl Pts',(-0.0315329431858092,1.8,1.));
#7966=CARTESIAN_POINT('Ctrl Pts',(-0.0650776639541239,1.79367084275751,
0.99835915024489));
#7967=CARTESIAN_POINT('Ctrl Pts',(-0.126634476150511,1.76811531482682,0.992431259450842));
#7968=CARTESIAN_POINT('Ctrl Pts',(-0.154657206767882,1.74889618382539,0.988223761669361));
#7969=CARTESIAN_POINT('Ctrl Pts',(-0.198899276956455,1.70465411363682,0.980277651290853));
#7970=CARTESIAN_POINT('Ctrl Pts',(-0.218115996279034,1.67663267125761,0.976011194447325));
#7971=CARTESIAN_POINT('Ctrl Pts',(-0.243669763522489,1.61508042700263,0.969947158664211));
#7972=CARTESIAN_POINT('Ctrl Pts',(-0.25,1.5815373526696,0.968245836551854));
#7973=CARTESIAN_POINT('Ctrl Pts',(-0.25,1.55,0.968245836551854));
#7974=CARTESIAN_POINT('',(-0.25,1.55,0.));
#7975=CARTESIAN_POINT('Origin',(1.65,2.25,0.));
#7976=CARTESIAN_POINT('',(-1.,2.25,-1.22464679914735E-16));
#7977=CARTESIAN_POINT('Origin',(0.,2.25,0.));
#7978=CARTESIAN_POINT('Origin',(1.75,0.85,0.));
#7979=CARTESIAN_POINT('',(-1.75,0.85,-2.14313189850787E-16));
#7980=CARTESIAN_POINT('Origin',(0.,0.85,0.));
#7981=CARTESIAN_POINT('Origin',(0.,0.,0.));
#7982=CARTESIAN_POINT('',(-1.75,-0.85,-2.14313189850787E-16));
#7983=CARTESIAN_POINT('Origin',(0.,-0.85,0.));
#7984=CARTESIAN_POINT('',(-1.75,0.,-2.14313189850787E-16));
#7985=CARTESIAN_POINT('Origin',(1.,-0.85,0.));
#7986=CARTESIAN_POINT('',(-1.,-0.85,-1.22464679914735E-16));
#7987=CARTESIAN_POINT('Origin',(0.,-0.85,0.));
#7988=CARTESIAN_POINT('Origin',(0.,0.7,0.));
#7989=CARTESIAN_POINT('',(-1.,0.7,-1.22464679914735E-16));
#9089=UNCERTAINTY_MEASURE_WITH_UNIT(LENGTH_MEASURE(0.001),#9142,
'DISTANCE_ACCURACY_VALUE',
'Maximum model space distance between geometric entities at asserted c
onnectivities');
#9108=UNCERTAINTY_MEASURE_WITH_UNIT(LENGTH_MEASURE(0.001),#9142,
'DISTANCE_ACCURACY_VALUE',
'Maximum model space distance between geometric entities at asserted c
onnectivities');
#9122=(
GEOMETRIC_REPRESENTATION_CONTEXT(3)
GLOBAL_UNCERTAINTY_ASSIGNED_CONTEXT((#9089))
GLOBAL_UNIT_ASSIGNED_CONTEXT((#9142,#9144,#9145))
REPRESENTATION_CONTEXT('','3D')
);
#9141=(
GEOMETRIC_REPRESENTATION_CONTEXT(3)
GLOBAL_UNCERTAINTY_ASSIGNED_CONTEXT((#9108))
GLOBAL_UNIT_ASSIGNED_CONTEXT((#9142,#9144,#9145))
REPRESENTATION_CONTEXT('','3D')
);
#9142=(
LENGTH_UNIT()
NAMED_UNIT(*)
SI_UNIT(.CENTI.,.METRE.)
);
#9144=(
NAMED_UNIT(*)
PLANE_ANGLE_UNIT()
SI_UNIT($,.RADIAN.)
);
#9145=(
NAMED_UNIT(*)
SI_UNIT($,.STERADIAN.)
SOLID_ANGLE_UNIT()
);
#9159=SHAPE_DEFINITION_REPRESENTATION(#9191,#9287);
#9191=PRODUCT_DEFINITION_SHAPE('',$,#9320);
#9287=SHAPE_REPRESENTATION('',(#5244),#9122);
#9306=PRODUCT_DEFINITION_CONTEXT('part definition',#9404,'design');
#9320=PRODUCT_DEFINITION('Insert bearing','Insert bearing',#9352,#9306);
#9352=PRODUCT_DEFINITION_FORMATION('',$,#9419);
#9404=APPLICATION_CONTEXT(
'Core Data for Automotive Mechanical Design Process');
#9405=PRODUCT_CONTEXT('part definition',#9404,'mechanical');
#9419=PRODUCT('Insert bearing','Insert bearing','Insert bearing',(#9405));
#9494=COLOUR_RGB('Grey',0.48,0.52,0.57);
#9495=FILL_AREA_STYLE_COLOUR('',#9494);
#9496=FILL_AREA_STYLE('',(#9495));
#9497=SURFACE_STYLE_FILL_AREA(#9496);
#9498=SURFACE_SIDE_STYLE('',(#9497));
#9499=SURFACE_STYLE_USAGE(.BOTH.,#9498);
#9500=PRESENTATION_STYLE_ASSIGNMENT((#9499));
ENDSEC;
END-ISO-10303-21;
